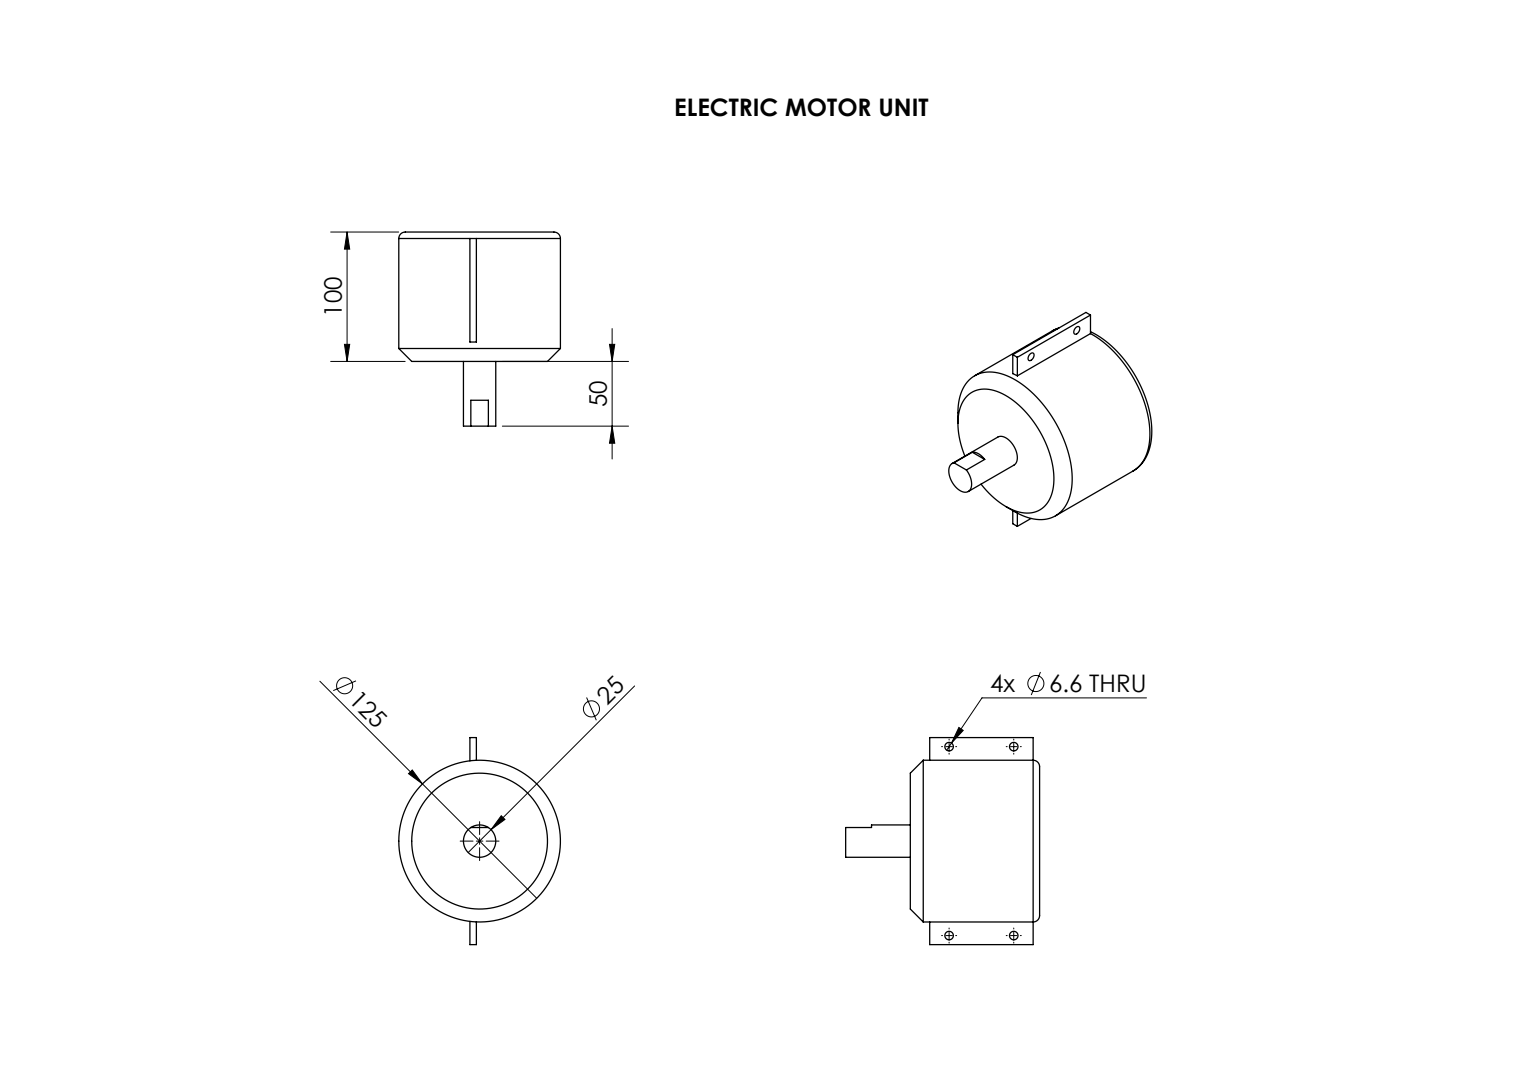
ISO-10303-21;
HEADER;
FILE_DESCRIPTION (('STEP AP214'),
    '1' );
FILE_NAME ('electric motor unit.step',
    '2026-10-08T09:53:37',
    ( '' ),
    ( '' ),
    'SwSTEP 2.0',
    'SolidWorks 2026',
    '' );
FILE_SCHEMA (( 'AUTOMOTIVE_DESIGN' ));
ENDSEC;

DATA;
#74=ORIENTED_EDGE ( 'NONE', *, *, #31039, .F. ) ;
#103=DIRECTION ( 'NONE',  ( 1.000000000000000000, 0.000000000000000000, 0.000000000000000000 ) ) ;
#302=ADVANCED_FACE ( 'NONE', ( #26021 ), #48946, .F. ) ;
#312=DIRECTION ( 'NONE',  ( 1.000000000000000000, 0.000000000000000000, -0.000000000000000000 ) ) ;
#361=ORIENTED_EDGE ( 'NONE', *, *, #62756, .T. ) ;
#411=EDGE_LOOP ( 'NONE', ( #54319, #60311, #25964, #66217 ) ) ;
#435=ORIENTED_EDGE ( 'NONE', *, *, #50527, .T. ) ;
#592=ORIENTED_EDGE ( 'NONE', *, *, #52648, .T. ) ;
#701=DIRECTION ( 'NONE',  ( -0.000000000000000000, -1.000000000000000000, -0.000000000000000000 ) ) ;
#748=DIRECTION ( 'NONE',  ( -2.628368902995175337E-16, -1.000000000000000000, 0.000000000000000000 ) ) ;
#850=LINE ( 'NONE', #68873, #20942 ) ;
#851=DIRECTION ( 'NONE',  ( 0.000000000000000000, 0.000000000000000000, -1.000000000000000000 ) ) ;
#862=ORIENTED_EDGE ( 'NONE', *, *, #52454, .F. ) ;
#988=ORIENTED_EDGE ( 'NONE', *, *, #17612, .T. ) ;
#1081=EDGE_CURVE ( 'NONE', #58897, #8861, #49235, .T. ) ;
#1100=DIRECTION ( 'NONE',  ( -1.000000000000000000, 0.000000000000000000, 0.000000000000000000 ) ) ;
#1101=ORIENTED_EDGE ( 'NONE', *, *, #21972, .F. ) ;
#1138=ORIENTED_EDGE ( 'NONE', *, *, #48438, .T. ) ;
#1246=VERTEX_POINT ( 'NONE', #31110 ) ;
#1350=CIRCLE ( 'NONE', #16923, 3.299999999999997158 ) ;
#1373=AXIS2_PLACEMENT_3D ( 'NONE', #24818, #13162, #19174 ) ;
#1428=EDGE_CURVE ( 'NONE', #19508, #17352, #18011, .T. ) ;
#1449=CARTESIAN_POINT ( 'NONE',  ( -57.50000000000000000, 0.000000000000000000, -270.0000000000000000 ) ) ;
#1479=FACE_OUTER_BOUND ( 'NONE', #30990, .T. ) ;
#1540=ORIENTED_EDGE ( 'NONE', *, *, #59533, .T. ) ;
#1570=CIRCLE ( 'NONE', #60360, 3.299999999999997158 ) ;
#1692=SURFACE_STYLE_FILL_AREA ( #25327 ) ;
#1812=DIRECTION ( 'NONE',  ( -1.000000000000000000, 0.000000000000000000, 0.000000000000000000 ) ) ;
#1846=CARTESIAN_POINT ( 'NONE',  ( -7.500000000000015099, -73.00000000000001421, -204.9999999999999716 ) ) ;
#1897=APPLICATION_CONTEXT ( 'automotive_design' ) ;
#1914=DIRECTION ( 'NONE',  ( 0.000000000000000000, -1.000000000000000000, 0.000000000000000000 ) ) ;
#1941=TOROIDAL_SURFACE ( 'NONE', #16270, 57.50000000000000000, 5.000000000000000000 ) ;
#2035=CLOSED_SHELL ( 'NONE', ( #30843, #53299, #302, #25026, #60112, #57640, #40573, #22486, #44929, #51198, #42095, #58290, #61829, #7482, #45373, #47263, #49888, #8489, #25397, #17549, #53469, #11560, #6297, #37604, #32650, #6641, #53402, #33495, #63872, #73659, #3012 ) ) ;
#2196=ORIENTED_EDGE ( 'NONE', *, *, #1428, .T. ) ;
#2277=ORIENTED_EDGE ( 'NONE', *, *, #3250, .T. ) ;
#2728=COLOUR_RGB ( '', 0.72549020, 0.75294118, 0.79215686) ;
#2822=DIRECTION ( 'NONE',  ( 1.000000000000000000, 0.000000000000000000, -0.000000000000000000 ) ) ;
#2995=ORIENTED_EDGE ( 'NONE', *, *, #17255, .F. ) ;
#3012=ADVANCED_FACE ( 'NONE', ( #22118 ), #14704, .F. ) ;
#3047=CARTESIAN_POINT ( 'NONE',  ( -2.500000000000015543, -73.00000000000001421, -255.0000000000000000 ) ) ;
#3250=EDGE_CURVE ( 'NONE', #46252, #45911, #14903, .T. ) ;
#3266=LINE ( 'NONE', #71272, #46651 ) ;
#3360=EDGE_CURVE ( 'NONE', #56357, #68556, #30997, .T. ) ;
#3614=ORIENTED_EDGE ( 'NONE', *, *, #35996, .T. ) ;
#3644=DIRECTION ( 'NONE',  ( 3.035766082959412415E-16, 1.000000000000000000, 0.000000000000000000 ) ) ;
#3658=AXIS2_PLACEMENT_3D ( 'NONE', #24375, #64239, #748 ) ;
#3682=CARTESIAN_POINT ( 'NONE',  ( -2.499999999999970690, 73.00000000000001421, -204.9999999999999716 ) ) ;
#3953=LINE ( 'NONE', #26854, #13909 ) ;
#3990=EDGE_CURVE ( 'NONE', #70803, #36870, #41096, .T. ) ;
#4050=DIRECTION ( 'NONE',  ( 1.000000000000000000, -3.035766082959412415E-16, 0.000000000000000000 ) ) ;
#4113=ORIENTED_EDGE ( 'NONE', *, *, #71182, .F. ) ;
#4170=EDGE_LOOP ( 'NONE', ( #2196, #10893 ) ) ;
#4251=ORIENTED_EDGE ( 'NONE', *, *, #46885, .T. ) ;
#4271=AXIS2_PLACEMENT_3D ( 'NONE', #41588, #29553, #64905 ) ;
#4350=ORIENTED_EDGE ( 'NONE', *, *, #62756, .F. ) ;
#4452=DIRECTION ( 'NONE',  ( -1.000000000000000000, 0.000000000000000000, -0.000000000000000000 ) ) ;
#4760=ORIENTED_EDGE ( 'NONE', *, *, #67736, .T. ) ;
#4846=ORIENTED_EDGE ( 'NONE', *, *, #59697, .F. ) ;
#4933=CIRCLE ( 'NONE', #1373, 62.50000000000000000 ) ;
#5052=AXIS2_PLACEMENT_3D ( 'NONE', #1449, #701, #36713 ) ;
#5114=DIRECTION ( 'NONE',  ( -3.035766082959412415E-16, -1.000000000000000000, -0.000000000000000000 ) ) ;
#5250=DIRECTION ( 'NONE',  ( -2.628368902995175337E-16, -1.000000000000000000, 0.000000000000000000 ) ) ;
#5361=AXIS2_PLACEMENT_3D ( 'NONE', #22738, #45676, #15965 ) ;
#5589=ORIENTED_EDGE ( 'NONE', *, *, #60526, .F. ) ;
#5681=DIRECTION ( 'NONE',  ( -2.628368902995175337E-16, -1.000000000000000000, 0.000000000000000000 ) ) ;
#5695=CARTESIAN_POINT ( 'NONE',  ( 62.50000000000000000, 0.000000000000000000, -184.9999999999999432 ) ) ;
#5706=FACE_OUTER_BOUND ( 'NONE', #38771, .T. ) ;
#5826=ORIENTED_EDGE ( 'NONE', *, *, #18491, .F. ) ;
#5919=FACE_OUTER_BOUND ( 'NONE', #16578, .T. ) ;
#5929=CARTESIAN_POINT ( 'NONE',  ( -62.50000000000000000, 7.654042494670957804E-15, -270.0000000000000000 ) ) ;
#6030=CARTESIAN_POINT ( 'NONE',  ( -7.500000000000015987, -76.30000000000001137, -204.9999999999999716 ) ) ;
#6194=LINE ( 'NONE', #16347, #44271 ) ;
#6210=VECTOR ( 'NONE', #10753, 1000.000000000000000 ) ;
#6241=DIRECTION ( 'NONE',  ( -1.000000000000000000, 0.000000000000000000, 0.000000000000000000 ) ) ;
#6297=ADVANCED_FACE ( 'NONE', ( #11593, #45473, #34534 ), #69492, .F. ) ;
#6395=CARTESIAN_POINT ( 'NONE',  ( -7.499999999999969802, 73.00000000000001421, -255.0000000000000000 ) ) ;
#6475=AXIS2_PLACEMENT_3D ( 'NONE', #28429, #40094, #32948 ) ;
#6550=CARTESIAN_POINT ( 'NONE',  ( 0.000000000000000000, 0.000000000000000000, -175.0000000000000000 ) ) ;
#6641=ADVANCED_FACE ( 'NONE', ( #72072, #33318, #39359 ), #21297, .T. ) ;
#6670=ORIENTED_EDGE ( 'NONE', *, *, #21705, .F. ) ;
#6743=EDGE_LOOP ( 'NONE', ( #46150, #36857 ) ) ;
#6818=DIRECTION ( 'NONE',  ( -1.000000000000000000, 0.000000000000000000, 0.000000000000000000 ) ) ;
#6845=EDGE_LOOP ( 'NONE', ( #46434, #7193 ) ) ;
#6891=CARTESIAN_POINT ( 'NONE',  ( -2.499999999999971578, 69.70000000000003126, -255.0000000000000000 ) ) ;
#7095=CIRCLE ( 'NONE', #23904, 3.299999999999983391 ) ;
#7161=AXIS2_PLACEMENT_3D ( 'NONE', #73193, #26956, #72082 ) ;
#7193=ORIENTED_EDGE ( 'NONE', *, *, #65149, .F. ) ;
#7283=AXIS2_PLACEMENT_3D ( 'NONE', #60970, #33494, #43696 ) ;
#7344=ORIENTED_EDGE ( 'NONE', *, *, #3250, .F. ) ;
#7449=DIRECTION ( 'NONE',  ( 1.000000000000000000, -3.061616997868382648E-16, -0.000000000000000000 ) ) ;
#7454=EDGE_CURVE ( 'NONE', #45911, #54824, #40915, .T. ) ;
#7482=ADVANCED_FACE ( 'NONE', ( #29600 ), #35312, .T. ) ;
#7679=LINE ( 'NONE', #53542, #74290 ) ;
#7748=VECTOR ( 'NONE', #42150, 1000.000000000000000 ) ;
#7797=CARTESIAN_POINT ( 'NONE',  ( -7.500000000000016875, -80.00000000000001421, -189.9999999999999147 ) ) ;
#7814=CARTESIAN_POINT ( 'NONE',  ( 6.782329983125270800, 10.49999999999999467, -145.0000000000000000 ) ) ;
#8026=SURFACE_SIDE_STYLE ('',( #1692 ) ) ;
#8037=AXIS2_PLACEMENT_3D ( 'NONE', #58333, #54183, #31232 ) ;
#8162=DIRECTION ( 'NONE',  ( -0.000000000000000000, -0.000000000000000000, -1.000000000000000000 ) ) ;
#8300=DIRECTION ( 'NONE',  ( 0.000000000000000000, 0.000000000000000000, -1.000000000000000000 ) ) ;
#8418=ORIENTED_EDGE ( 'NONE', *, *, #21972, .T. ) ;
#8489=ADVANCED_FACE ( 'NONE', ( #31932 ), #60891, .F. ) ;
#8518=CIRCLE ( 'NONE', #44539, 3.299999999999983391 ) ;
#8603=( NAMED_UNIT ( * ) SI_UNIT ( $, .STERADIAN. ) SOLID_ANGLE_UNIT ( ) );
#8735=EDGE_CURVE ( 'NONE', #28195, #41791, #63793, .T. ) ;
#8755=EDGE_CURVE ( 'NONE', #43515, #60602, #68396, .T. ) ;
#8796=LINE ( 'NONE', #31713, #23348 ) ;
#8861=VERTEX_POINT ( 'NONE', #69850 ) ;
#8895=CARTESIAN_POINT ( 'NONE',  ( -7.499999999999969802, 76.30000000000001137, -204.9999999999999716 ) ) ;
#8926=CARTESIAN_POINT ( 'NONE',  ( -7.500000000000011546, -62.04836822995428491, -270.0000000000000000 ) ) ;
#8965=( NAMED_UNIT ( * ) SI_UNIT ( $, .STERADIAN. ) SOLID_ANGLE_UNIT ( ) );
#9003=VECTOR ( 'NONE', #20553, 1000.000000000000000 ) ;
#9296=ORIENTED_EDGE ( 'NONE', *, *, #25138, .F. ) ;
#9298=CYLINDRICAL_SURFACE ( 'NONE', #7161, 3.299999999999983391 ) ;
#9305=CARTESIAN_POINT ( 'NONE',  ( -7.500000000000015987, -76.29999999999999716, -255.0000000000000000 ) ) ;
#9325=SHAPE_REPRESENTATION_RELATIONSHIP ( 'NONE' , 'NONE' ,  #72820, #21132 ) ;
#9442=LINE ( 'NONE', #19610, #22727 ) ;
#9750=DIRECTION ( 'NONE',  ( -0.7071067811865485719, 0.000000000000000000, -0.7071067811865465735 ) ) ;
#9822=ORIENTED_EDGE ( 'NONE', *, *, #23184, .T. ) ;
#9848=AXIS2_PLACEMENT_3D ( 'NONE', #39904, #17697, #63579 ) ;
#10049=CARTESIAN_POINT ( 'NONE',  ( 0.000000000000000000, 0.000000000000000000, -275.0000000000000000 ) ) ;
#10147=ORIENTED_EDGE ( 'NONE', *, *, #43144, .F. ) ;
#10415=ORIENTED_EDGE ( 'NONE', *, *, #54147, .T. ) ;
#10450=CIRCLE ( 'NONE', #8037, 52.50000000000002132 ) ;
#10569=FACE_OUTER_BOUND ( 'NONE', #62660, .T. ) ;
#10575=VECTOR ( 'NONE', #5114, 1000.000000000000000 ) ;
#10601=AXIS2_PLACEMENT_3D ( 'NONE', #13781, #59665, #20550 ) ;
#10656=CARTESIAN_POINT ( 'NONE',  ( 12.49999999999999645, 0.000000000000000000, -175.0000000000000000 ) ) ;
#10753=DIRECTION ( 'NONE',  ( -0.000000000000000000, -0.000000000000000000, 1.000000000000000000 ) ) ;
#10867=UNCERTAINTY_MEASURE_WITH_UNIT (LENGTH_MEASURE( 1.000000000000000082E-05 ), #72476, 'distance_accuracy_value', 'NONE');
#10893=ORIENTED_EDGE ( 'NONE', *, *, #27823, .T. ) ;
#10996=PLANE ( 'NONE',  #14198 ) ;
#11029=CIRCLE ( 'NONE', #18269, 3.299999999999997158 ) ;
#11050=ORIENTED_EDGE ( 'NONE', *, *, #64960, .F. ) ;
#11195=DIRECTION ( 'NONE',  ( 2.628368902995164490E-16, 1.000000000000000000, 0.000000000000000000 ) ) ;
#11360=EDGE_CURVE ( 'NONE', #60498, #28566, #43303, .T. ) ;
#11393=ORIENTED_EDGE ( 'NONE', *, *, #11360, .F. ) ;
#11528=CARTESIAN_POINT ( 'NONE',  ( 0.000000000000000000, 0.000000000000000000, -275.0000000000000000 ) ) ;
#11552=DIRECTION ( 'NONE',  ( 1.000000000000000000, -3.061616997868382648E-16, -0.000000000000000000 ) ) ;
#11560=ADVANCED_FACE ( 'NONE', ( #26385, #43337, #10569 ), #49312, .T. ) ;
#11575=CARTESIAN_POINT ( 'NONE',  ( -62.50000000000000000, 7.654042494670957804E-15, -184.9999999999999432 ) ) ;
#11593=FACE_BOUND ( 'NONE', #62231, .T. ) ;
#11635=ORIENTED_EDGE ( 'NONE', *, *, #12276, .T. ) ;
#11806=EDGE_CURVE ( 'NONE', #65637, #48516, #4933, .T. ) ;
#11844=FACE_OUTER_BOUND ( 'NONE', #29116, .T. ) ;
#11924=VECTOR ( 'NONE', #71334, 1000.000000000000000 ) ;
#12094=ORIENTED_EDGE ( 'NONE', *, *, #7454, .T. ) ;
#12148=CARTESIAN_POINT ( 'NONE',  ( -7.500000000000015099, -73.00000000000001421, -204.9999999999999716 ) ) ;
#12276=EDGE_CURVE ( 'NONE', #59175, #17352, #47770, .T. ) ;
#12340=DIRECTION ( 'NONE',  ( 2.628368902995164490E-16, 1.000000000000000000, 0.000000000000000000 ) ) ;
#12550=( NAMED_UNIT ( * ) PLANE_ANGLE_UNIT ( ) SI_UNIT ( $, .RADIAN. ) );
#12573=ORIENTED_EDGE ( 'NONE', *, *, #1081, .F. ) ;
#12621=AXIS2_PLACEMENT_3D ( 'NONE', #51765, #58509, #312 ) ;
#12671=ORIENTED_EDGE ( 'NONE', *, *, #16152, .T. ) ;
#12691=CARTESIAN_POINT ( 'NONE',  ( 0.000000000000000000, 0.000000000000000000, -184.9999999999999432 ) ) ;
#13153=AXIS2_PLACEMENT_3D ( 'NONE', #24806, #70649, #37211 ) ;
#13162=DIRECTION ( 'NONE',  ( -0.000000000000000000, -0.000000000000000000, -1.000000000000000000 ) ) ;
#13218=EDGE_CURVE ( 'NONE', #20502, #14677, #59869, .T. ) ;
#13293=( LENGTH_UNIT ( ) NAMED_UNIT ( * ) SI_UNIT ( .MILLI., .METRE. ) );
#13320=CARTESIAN_POINT ( 'NONE',  ( -2.500000000000014655, -69.70000000000003126, -255.0000000000000000 ) ) ;
#13374=AXIS2_PLACEMENT_3D ( 'NONE', #55982, #49591, #26291 ) ;
#13556=LINE ( 'NONE', #36861, #7748 ) ;
#13587=AXIS2_PLACEMENT_3D ( 'NONE', #45939, #69592, #33899 ) ;
#13620=ORIENTED_EDGE ( 'NONE', *, *, #17255, .T. ) ;
#13781=CARTESIAN_POINT ( 'NONE',  ( 0.000000000000000000, 0.000000000000000000, -270.0000000000000000 ) ) ;
#13845=AXIS2_PLACEMENT_3D ( 'NONE', #10049, #14577, #38252 ) ;
#13848=SURFACE_STYLE_FILL_AREA ( #72108 ) ;
#13872=ORIENTED_EDGE ( 'NONE', *, *, #25138, .T. ) ;
#13909=VECTOR ( 'NONE', #27211, 1000.000000000000000 ) ;
#14112=ORIENTED_EDGE ( 'NONE', *, *, #31568, .F. ) ;
#14114=AXIS2_PLACEMENT_3D ( 'NONE', #66883, #60158, #31549 ) ;
#14129=ORIENTED_EDGE ( 'NONE', *, *, #52454, .T. ) ;
#14164=ORIENTED_EDGE ( 'NONE', *, *, #1081, .T. ) ;
#14198=AXIS2_PLACEMENT_3D ( 'NONE', #21899, #33168, #16258 ) ;
#14261=PLANE ( 'NONE',  #13153 ) ;
#14402=PLANE ( 'NONE',  #69131 ) ;
#14414=ORIENTED_EDGE ( 'NONE', *, *, #46092, .T. ) ;
#14577=DIRECTION ( 'NONE',  ( 0.000000000000000000, 0.000000000000000000, -1.000000000000000000 ) ) ;
#14677=VERTEX_POINT ( 'NONE', #49938 ) ;
#14704=CYLINDRICAL_SURFACE ( 'NONE', #27337, 3.299999999999983391 ) ;
#14826=CARTESIAN_POINT ( 'NONE',  ( 0.000000000000000000, 0.000000000000000000, -270.0000000000000000 ) ) ;
#14903=LINE ( 'NONE', #54027, #59829 ) ;
#14969=CARTESIAN_POINT ( 'NONE',  ( -7.500000000000016875, -80.00000000000001421, -189.9999999999999147 ) ) ;
#15362=ORIENTED_EDGE ( 'NONE', *, *, #21277, .F. ) ;
#15420=ORIENTED_EDGE ( 'NONE', *, *, #53796, .F. ) ;
#15467=CYLINDRICAL_SURFACE ( 'NONE', #47896, 12.49999999999999645 ) ;
#15499=VERTEX_POINT ( 'NONE', #5929 ) ;
#15513=ORIENTED_EDGE ( 'NONE', *, *, #64442, .T. ) ;
#15807=CIRCLE ( 'NONE', #9848, 12.49999999999999645 ) ;
#15965=DIRECTION ( 'NONE',  ( -1.000000000000000000, 0.000000000000000000, 0.000000000000000000 ) ) ;
#16108=VERTEX_POINT ( 'NONE', #29746 ) ;
#16152=EDGE_CURVE ( 'NONE', #41791, #67978, #53077, .T. ) ;
#16239=ORIENTED_EDGE ( 'NONE', *, *, #8755, .F. ) ;
#16252=ORIENTED_EDGE ( 'NONE', *, *, #45421, .T. ) ;
#16258=DIRECTION ( 'NONE',  ( 3.035766082959412415E-16, 1.000000000000000000, 0.000000000000000000 ) ) ;
#16270=AXIS2_PLACEMENT_3D ( 'NONE', #58457, #64118, #6241 ) ;
#16310=MECHANICAL_DESIGN_GEOMETRIC_PRESENTATION_REPRESENTATION('',(#28319),#59517);
#16347=CARTESIAN_POINT ( 'NONE',  ( -7.499999999999968914, 79.99999999999998579, -269.9999999999999432 ) ) ;
#16355=EDGE_LOOP ( 'NONE', ( #22088, #592, #74262, #11050 ) ) ;
#16369=CARTESIAN_POINT ( 'NONE',  ( -2.500000000000017319, -80.00000000000001421, -269.9999999999999432 ) ) ;
#16373=DIRECTION ( 'NONE',  ( -2.628368902995175337E-16, -1.000000000000000000, 0.000000000000000000 ) ) ;
#16391=CARTESIAN_POINT ( 'NONE',  ( -62.50000000000000000, 7.654042494670957804E-15, -275.0000000000000000 ) ) ;
#16486=ORIENTED_EDGE ( 'NONE', *, *, #59697, .T. ) ;
#16494=ORIENTED_EDGE ( 'NONE', *, *, #19258, .T. ) ;
#16557=VERTEX_POINT ( 'NONE', #53348 ) ;
#16578=EDGE_LOOP ( 'NONE', ( #54271, #65011, #23966, #27736, #3614, #65107, #26363, #21177 ) ) ;
#16725=ORIENTED_EDGE ( 'NONE', *, *, #57755, .T. ) ;
#16923=AXIS2_PLACEMENT_3D ( 'NONE', #3682, #71692, #26944 ) ;
#17255=EDGE_CURVE ( 'NONE', #67978, #16108, #38669, .T. ) ;
#17304=AXIS2_PLACEMENT_3D ( 'NONE', #37039, #72353, #36289 ) ;
#17339=CYLINDRICAL_SURFACE ( 'NONE', #25457, 62.50000000000000000 ) ;
#17347=DIRECTION ( 'NONE',  ( -1.000000000000000000, -3.907985046680551022E-14, 0.000000000000000000 ) ) ;
#17352=VERTEX_POINT ( 'NONE', #68636 ) ;
#17357=DIRECTION ( 'NONE',  ( -3.035766082959412415E-16, -1.000000000000000000, -0.000000000000000000 ) ) ;
#17395=PRODUCT_CONTEXT ( 'NONE', #29621, 'mechanical' ) ;
#17544=CYLINDRICAL_SURFACE ( 'NONE', #66014, 62.50000000000000000 ) ;
#17549=ADVANCED_FACE ( 'NONE', ( #25353 ), #43406, .F. ) ;
#17612=EDGE_CURVE ( 'NONE', #28566, #28744, #8796, .T. ) ;
#17697=DIRECTION ( 'NONE',  ( 0.000000000000000000, 0.000000000000000000, 1.000000000000000000 ) ) ;
#17702=VECTOR ( 'NONE', #44493, 1000.000000000000000 ) ;
#17760=CARTESIAN_POINT ( 'NONE',  ( 0.000000000000000000, 0.000000000000000000, -189.9999999999999147 ) ) ;
#17773=CARTESIAN_POINT ( 'NONE',  ( -7.499999999999968914, 79.99999999999998579, -189.9999999999999147 ) ) ;
#17824=CARTESIAN_POINT ( 'NONE',  ( -2.499999999999974243, 62.44997998398397954, -275.0000000000000000 ) ) ;
#17827=CIRCLE ( 'NONE', #27423, 62.50000000000000000 ) ;
#17921=FACE_OUTER_BOUND ( 'NONE', #31873, .T. ) ;
#18011=CIRCLE ( 'NONE', #51603, 57.50000000000000000 ) ;
#18018=VECTOR ( 'NONE', #8300, 1000.000000000000000 ) ;
#18112=CARTESIAN_POINT ( 'NONE',  ( -7.500000000000015099, -73.00000000000001421, -255.0000000000000000 ) ) ;
#18269=AXIS2_PLACEMENT_3D ( 'NONE', #54497, #19534, #42486 ) ;
#18314=AXIS2_PLACEMENT_3D ( 'NONE', #14826, #32111, #42668 ) ;
#18316=DIRECTION ( 'NONE',  ( -0.000000000000000000, -0.000000000000000000, 1.000000000000000000 ) ) ;
#18420=ORIENTED_EDGE ( 'NONE', *, *, #67960, .T. ) ;
#18491=EDGE_CURVE ( 'NONE', #1246, #39261, #44228, .T. ) ;
#18590=LINE ( 'NONE', #23500, #22811 ) ;
#18630=AXIS2_PLACEMENT_3D ( 'NONE', #73390, #66658, #73011 ) ;
#18638=VECTOR ( 'NONE', #66465, 1000.000000000000000 ) ;
#18647=CYLINDRICAL_SURFACE ( 'NONE', #4271, 3.299999999999997158 ) ;
#18827=CARTESIAN_POINT ( 'NONE',  ( -2.500000000000017319, -80.00000000000001421, -189.9999999999999147 ) ) ;
#18845=VECTOR ( 'NONE', #9750, 1000.000000000000000 ) ;
#18974=EDGE_LOOP ( 'NONE', ( #57902, #37363, #12573, #43298 ) ) ;
#19154=CARTESIAN_POINT ( 'NONE',  ( -6.782329983125270800, 10.49999999999999467, -145.0000000000000000 ) ) ;
#19174=DIRECTION ( 'NONE',  ( -1.000000000000000000, 0.000000000000000000, 0.000000000000000000 ) ) ;
#19206=LINE ( 'NONE', #59813, #18018 ) ;
#19258=EDGE_CURVE ( 'NONE', #45911, #70771, #63294, .T. ) ;
#19508=VERTEX_POINT ( 'NONE', #42434 ) ;
#19534=DIRECTION ( 'NONE',  ( -1.000000000000000000, 3.061616997868382648E-16, 0.000000000000000000 ) ) ;
#19555=DIRECTION ( 'NONE',  ( -1.000000000000000000, 3.061616997868382648E-16, 0.000000000000000000 ) ) ;
#19573=ORIENTED_EDGE ( 'NONE', *, *, #23372, .F. ) ;
#19610=CARTESIAN_POINT ( 'NONE',  ( -7.499999999999969802, 76.30000000000001137, -204.9999999999999716 ) ) ;
#19636=CARTESIAN_POINT ( 'NONE',  ( -2.499999999999970690, 73.00000000000001421, -255.0000000000000000 ) ) ;
#19735=DIRECTION ( 'NONE',  ( 1.000000000000000000, 0.000000000000000000, 0.000000000000000000 ) ) ;
#19847=ORIENTED_EDGE ( 'NONE', *, *, #63123, .F. ) ;
#20050=VERTEX_POINT ( 'NONE', #52720 ) ;
#20152=CARTESIAN_POINT ( 'NONE',  ( -2.500000000000011990, -62.44997998398397954, -269.9999999999999432 ) ) ;
#20172=ORIENTED_EDGE ( 'NONE', *, *, #54847, .T. ) ;
#20393=DIRECTION ( 'NONE',  ( 1.000000000000000000, -3.061616997868382648E-16, -0.000000000000000000 ) ) ;
#20502=VERTEX_POINT ( 'NONE', #52529 ) ;
#20550=DIRECTION ( 'NONE',  ( -1.000000000000000000, 0.000000000000000000, 0.000000000000000000 ) ) ;
#20553=DIRECTION ( 'NONE',  ( -0.000000000000000000, -0.000000000000000000, 1.000000000000000000 ) ) ;
#20568=ORIENTED_EDGE ( 'NONE', *, *, #3990, .T. ) ;
#20596=LINE ( 'NONE', #43547, #18638 ) ;
#20796=EDGE_CURVE ( 'NONE', #15499, #65637, #67901, .T. ) ;
#20847=CIRCLE ( 'NONE', #6475, 62.50000000000000000 ) ;
#20942=VECTOR ( 'NONE', #17357, 1000.000000000000000 ) ;
#21132=ADVANCED_BREP_SHAPE_REPRESENTATION ( '', ( #37419, #43395 ), #41132 ) ;
#21177=ORIENTED_EDGE ( 'NONE', *, *, #50081, .T. ) ;
#21277=EDGE_CURVE ( 'NONE', #20050, #32222, #11029, .T. ) ;
#21297=PLANE ( 'NONE',  #56843 ) ;
#21436=ORIENTED_EDGE ( 'NONE', *, *, #54640, .F. ) ;
#21442=LINE ( 'NONE', #73322, #49807 ) ;
#21668=EDGE_CURVE ( 'NONE', #15499, #56357, #68728, .T. ) ;
#21673=FACE_BOUND ( 'NONE', #25864, .T. ) ;
#21702=AXIS2_PLACEMENT_3D ( 'NONE', #19154, #1914, #58641 ) ;
#21705=EDGE_CURVE ( 'NONE', #59850, #48671, #1570, .T. ) ;
#21786=PRODUCT_DEFINITION_SHAPE ( 'NONE', 'NONE',  #33419 ) ;
#21797=CIRCLE ( 'NONE', #48215, 3.299999999999997158 ) ;
#21899=CARTESIAN_POINT ( 'NONE',  ( -7.499999999999992895, 2.289750019674042456E-15, 0.000000000000000000 ) ) ;
#21972=EDGE_CURVE ( 'NONE', #41089, #33185, #21797, .T. ) ;
#21988=LINE ( 'NONE', #17824, #44781 ) ;
#21996=EDGE_CURVE ( 'NONE', #16108, #67978, #43405, .T. ) ;
#22060=CARTESIAN_POINT ( 'NONE',  ( -2.499999999999992895, 7.589415207398510330E-16, 0.000000000000000000 ) ) ;
#22088=ORIENTED_EDGE ( 'NONE', *, *, #21705, .T. ) ;
#22118=FACE_OUTER_BOUND ( 'NONE', #46049, .T. ) ;
#22371=ORIENTED_EDGE ( 'NONE', *, *, #42422, .F. ) ;
#22486=ADVANCED_FACE ( 'NONE', ( #5706 ), #17339, .T. ) ;
#22649=FACE_OUTER_BOUND ( 'NONE', #60918, .T. ) ;
#22705=ORIENTED_EDGE ( 'NONE', *, *, #37349, .F. ) ;
#22727=VECTOR ( 'NONE', #31998, 1000.000000000000000 ) ;
#22738=CARTESIAN_POINT ( 'NONE',  ( 0.000000000000000000, 0.000000000000000000, -184.9999999999999432 ) ) ;
#22799=CARTESIAN_POINT ( 'NONE',  ( -7.500000000000014211, -69.70000000000001705, -204.9999999999999716 ) ) ;
#22811=VECTOR ( 'NONE', #46813, 1000.000000000000000 ) ;
#22862=CYLINDRICAL_SURFACE ( 'NONE', #37805, 3.299999999999997158 ) ;
#22866=EDGE_CURVE ( 'NONE', #60498, #65293, #35637, .T. ) ;
#23017=VECTOR ( 'NONE', #3644, 1000.000000000000000 ) ;
#23019=CARTESIAN_POINT ( 'NONE',  ( 0.000000000000000000, 0.000000000000000000, -125.0000000000000000 ) ) ;
#23184=EDGE_CURVE ( 'NONE', #71821, #24035, #55552, .T. ) ;
#23348=VECTOR ( 'NONE', #54658, 1000.000000000000000 ) ;
#23372=EDGE_CURVE ( 'NONE', #40539, #62152, #21988, .T. ) ;
#23380=CIRCLE ( 'NONE', #59436, 12.49999999999999645 ) ;
#23489=VERTEX_POINT ( 'NONE', #28735 ) ;
#23500=CARTESIAN_POINT ( 'NONE',  ( 62.50000000000000000, 7.654042494670957804E-15, -184.9999999999999432 ) ) ;
#23523=DIRECTION ( 'NONE',  ( 0.000000000000000000, 0.000000000000000000, -1.000000000000000000 ) ) ;
#23728=ORIENTED_EDGE ( 'NONE', *, *, #73905, .T. ) ;
#23904=AXIS2_PLACEMENT_3D ( 'NONE', #3047, #19555, #65072 ) ;
#23939=PLANE ( 'NONE',  #12621 ) ;
#23966=ORIENTED_EDGE ( 'NONE', *, *, #45421, .F. ) ;
#24035=VERTEX_POINT ( 'NONE', #43189 ) ;
#24075=DIRECTION ( 'NONE',  ( -1.000000000000000000, 0.000000000000000000, 0.000000000000000000 ) ) ;
#24215=DIRECTION ( 'NONE',  ( 0.000000000000000000, 0.000000000000000000, -1.000000000000000000 ) ) ;
#24375=CARTESIAN_POINT ( 'NONE',  ( -2.500000000000015543, -73.00000000000001421, -255.0000000000000000 ) ) ;
#24537=CARTESIAN_POINT ( 'NONE',  ( -7.499999999999970690, 69.70000000000003126, -255.0000000000000000 ) ) ;
#24770=LINE ( 'NONE', #53711, #26325 ) ;
#24806=CARTESIAN_POINT ( 'NONE',  ( -7.500000000000016875, -80.00000000000001421, -269.9999999999999432 ) ) ;
#24818=CARTESIAN_POINT ( 'NONE',  ( 0.000000000000000000, 0.000000000000000000, -184.9999999999999432 ) ) ;
#24821=LINE ( 'NONE', #64679, #73542 ) ;
#24907=DIRECTION ( 'NONE',  ( -1.000000000000000000, 0.000000000000000000, 0.000000000000000000 ) ) ;
#24967=ORIENTED_EDGE ( 'NONE', *, *, #46092, .F. ) ;
#25026=ADVANCED_FACE ( 'NONE', ( #30405 ), #41335, .F. ) ;
#25138=EDGE_CURVE ( 'NONE', #59175, #40539, #65382, .T. ) ;
#25158=CARTESIAN_POINT ( 'NONE',  ( 0.000000000000000000, 0.000000000000000000, -270.0000000000000000 ) ) ;
#25327=FILL_AREA_STYLE ('',( #59915 ) ) ;
#25353=FACE_OUTER_BOUND ( 'NONE', #32700, .T. ) ;
#25397=ADVANCED_FACE ( 'NONE', ( #40140 ), #22862, .F. ) ;
#25457=AXIS2_PLACEMENT_3D ( 'NONE', #28604, #63591, #103 ) ;
#25565=UNCERTAINTY_MEASURE_WITH_UNIT (LENGTH_MEASURE( 1.000000000000000082E-05 ), #13293, 'distance_accuracy_value', 'NONE');
#25708=DIRECTION ( 'NONE',  ( 0.000000000000000000, 0.000000000000000000, 1.000000000000000000 ) ) ;
#25752=DIRECTION ( 'NONE',  ( 3.035766082959412415E-16, 1.000000000000000000, 0.000000000000000000 ) ) ;
#25800=CARTESIAN_POINT ( 'NONE',  ( -7.500000000000016875, -80.00000000000001421, -189.9999999999999147 ) ) ;
#25845=PRODUCT_DEFINITION_CONTEXT ( 'detailed design', #1897, 'design' ) ;
#25864=EDGE_LOOP ( 'NONE', ( #26166, #16725 ) ) ;
#25880=SURFACE_STYLE_USAGE ( .BOTH. , #37913 ) ;
#25964=ORIENTED_EDGE ( 'NONE', *, *, #42422, .T. ) ;
#26021=FACE_OUTER_BOUND ( 'NONE', #16355, .T. ) ;
#26089=AXIS2_PLACEMENT_3D ( 'NONE', #37500, #32939, #49863 ) ;
#26166=ORIENTED_EDGE ( 'NONE', *, *, #11360, .T. ) ;
#26254=ORIENTED_EDGE ( 'NONE', *, *, #72617, .F. ) ;
#26291=DIRECTION ( 'NONE',  ( 2.628368902995175337E-16, 1.000000000000000000, 0.000000000000000000 ) ) ;
#26325=VECTOR ( 'NONE', #30763, 1000.000000000000000 ) ;
#26363=ORIENTED_EDGE ( 'NONE', *, *, #58415, .T. ) ;
#26385=FACE_BOUND ( 'NONE', #29466, .T. ) ;
#26431=CIRCLE ( 'NONE', #63646, 3.299999999999983391 ) ;
#26613=PLANE ( 'NONE',  #41903 ) ;
#26652=EDGE_LOOP ( 'NONE', ( #37636, #43197, #7344, #55793 ) ) ;
#26697=ORIENTED_EDGE ( 'NONE', *, *, #46618, .T. ) ;
#26854=CARTESIAN_POINT ( 'NONE',  ( -7.500000000000014211, -69.70000000000003126, -255.0000000000000000 ) ) ;
#26921=DIRECTION ( 'NONE',  ( -1.000000000000000000, 0.000000000000000000, 0.000000000000000000 ) ) ;
#26944=DIRECTION ( 'NONE',  ( -2.628368902995164490E-16, -1.000000000000000000, 0.000000000000000000 ) ) ;
#26956=DIRECTION ( 'NONE',  ( 1.000000000000000000, -3.061616997868382648E-16, -0.000000000000000000 ) ) ;
#27053=EDGE_LOOP ( 'NONE', ( #4251, #32061 ) ) ;
#27108=AXIS2_PLACEMENT_3D ( 'NONE', #23019, #851, #45948 ) ;
#27148=PLANE ( 'NONE',  #18630 ) ;
#27211=DIRECTION ( 'NONE',  ( 1.000000000000000000, -3.061616997868382648E-16, -0.000000000000000000 ) ) ;
#27329=FACE_OUTER_BOUND ( 'NONE', #4170, .T. ) ;
#27337=AXIS2_PLACEMENT_3D ( 'NONE', #54930, #27756, #50303 ) ;
#27374=ORIENTED_EDGE ( 'NONE', *, *, #11806, .F. ) ;
#27423=AXIS2_PLACEMENT_3D ( 'NONE', #45937, #68861, #17347 ) ;
#27549=LINE ( 'NONE', #38471, #17702 ) ;
#27736=ORIENTED_EDGE ( 'NONE', *, *, #59261, .F. ) ;
#27756=DIRECTION ( 'NONE',  ( 1.000000000000000000, -3.061616997868382648E-16, -0.000000000000000000 ) ) ;
#27787=CARTESIAN_POINT ( 'NONE',  ( -7.499999999999969802, 73.00000000000001421, -255.0000000000000000 ) ) ;
#27802=CARTESIAN_POINT ( 'NONE',  ( -7.499999999999968914, 79.99999999999998579, -189.9999999999999147 ) ) ;
#27823=EDGE_CURVE ( 'NONE', #17352, #19508, #34525, .T. ) ;
#27977=CARTESIAN_POINT ( 'NONE',  ( -2.500000000000011990, -62.44997998398397954, -275.0000000000000000 ) ) ;
#28016=DIRECTION ( 'NONE',  ( -1.000000000000000000, 1.776356839400250465E-15, 0.000000000000000000 ) ) ;
#28195=VERTEX_POINT ( 'NONE', #33974 ) ;
#28319=STYLED_ITEM ( 'NONE', ( #53891 ), #37419 ) ;
#28346=LINE ( 'NONE', #27977, #43472 ) ;
#28429=CARTESIAN_POINT ( 'NONE',  ( 0.000000000000000000, 0.000000000000000000, -184.9999999999999432 ) ) ;
#28516=DIRECTION ( 'NONE',  ( 1.000000000000000000, -3.061616997868382648E-16, -0.000000000000000000 ) ) ;
#28566=VERTEX_POINT ( 'NONE', #61723 ) ;
#28604=CARTESIAN_POINT ( 'NONE',  ( 0.000000000000000000, 0.000000000000000000, -275.0000000000000000 ) ) ;
#28635=DIRECTION ( 'NONE',  ( -1.000000000000000000, 0.000000000000000000, -0.000000000000000000 ) ) ;
#28735=CARTESIAN_POINT ( 'NONE',  ( -52.50000000000002132, 0.000000000000000000, -175.0000000000000000 ) ) ;
#28744=VERTEX_POINT ( 'NONE', #52286 ) ;
#28774=EDGE_CURVE ( 'NONE', #36870, #60602, #46649, .T. ) ;
#28783=CIRCLE ( 'NONE', #34745, 52.50000000000002132 ) ;
#28903=CARTESIAN_POINT ( 'NONE',  ( 12.49999999999999645, 0.000000000000000000, -175.0000000000000000 ) ) ;
#28955=DIRECTION ( 'NONE',  ( 0.000000000000000000, 0.000000000000000000, -1.000000000000000000 ) ) ;
#29116=EDGE_LOOP ( 'NONE', ( #9296, #11635, #56965, #21436, #24967, #74072 ) ) ;
#29327=ORIENTED_EDGE ( 'NONE', *, *, #35996, .F. ) ;
#29466=EDGE_LOOP ( 'NONE', ( #60592, #13620 ) ) ;
#29553=DIRECTION ( 'NONE',  ( 1.000000000000000000, -3.061616997868382648E-16, -0.000000000000000000 ) ) ;
#29600=FACE_OUTER_BOUND ( 'NONE', #53704, .T. ) ;
#29618=DIRECTION ( 'NONE',  ( 3.035766082959412415E-16, 1.000000000000000000, 0.000000000000000000 ) ) ;
#29621=APPLICATION_CONTEXT ( 'automotive_design' ) ;
#29683=CARTESIAN_POINT ( 'NONE',  ( 12.49999999999999645, 0.000000000000000000, -125.0000000000000000 ) ) ;
#29746=CARTESIAN_POINT ( 'NONE',  ( -2.499999999999969802, 76.29999999999999716, -255.0000000000000000 ) ) ;
#29765=SHAPE_DEFINITION_REPRESENTATION ( #21786, #72820 ) ;
#30194=EDGE_CURVE ( 'NONE', #40539, #40791, #17827, .T. ) ;
#30255=CARTESIAN_POINT ( 'NONE',  ( -7.500000000000016875, -80.00000000000001421, -269.9999999999999432 ) ) ;
#30270=EDGE_CURVE ( 'NONE', #8861, #58897, #7095, .T. ) ;
#30329=AXIS2_PLACEMENT_3D ( 'NONE', #19636, #59507, #47843 ) ;
#30405=FACE_OUTER_BOUND ( 'NONE', #63386, .T. ) ;
#30478=LINE ( 'NONE', #18827, #39541 ) ;
#30502=EDGE_LOOP ( 'NONE', ( #45891, #26697, #62164, #2995 ) ) ;
#30520=VECTOR ( 'NONE', #59680, 1000.000000000000000 ) ;
#30763=DIRECTION ( 'NONE',  ( -0.000000000000000000, -0.000000000000000000, 1.000000000000000000 ) ) ;
#30843=ADVANCED_FACE ( 'NONE', ( #67192 ), #9298, .F. ) ;
#30931=ORIENTED_EDGE ( 'NONE', *, *, #43144, .T. ) ;
#30990=EDGE_LOOP ( 'NONE', ( #1138, #10415 ) ) ;
#30997=CIRCLE ( 'NONE', #10601, 62.50000000000000000 ) ;
#31028=VECTOR ( 'NONE', #52655, 1000.000000000000000 ) ;
#31039=EDGE_CURVE ( 'NONE', #46252, #16557, #48294, .T. ) ;
#31110=CARTESIAN_POINT ( 'NONE',  ( -6.782329983125270800, 10.49999999999999467, -145.0000000000000000 ) ) ;
#31232=DIRECTION ( 'NONE',  ( -1.000000000000000000, 0.000000000000000000, 0.000000000000000000 ) ) ;
#31233=AXIS2_PLACEMENT_3D ( 'NONE', #1846, #7449, #12340 ) ;
#31549=DIRECTION ( 'NONE',  ( -1.000000000000000000, 0.000000000000000000, 0.000000000000000000 ) ) ;
#31568=EDGE_CURVE ( 'NONE', #45157, #65293, #66739, .T. ) ;
#31582=CARTESIAN_POINT ( 'NONE',  ( -2.500000000000017319, -80.00000000000001421, -189.9999999999999147 ) ) ;
#31618=ORIENTED_EDGE ( 'NONE', *, *, #50081, .F. ) ;
#31713=CARTESIAN_POINT ( 'NONE',  ( -12.49999999999999645, 1.530808498934191127E-15, -175.0000000000000000 ) ) ;
#31832=CIRCLE ( 'NONE', #34256, 12.49999999999999645 ) ;
#31833=EDGE_LOOP ( 'NONE', ( #29327, #49092, #19847, #862 ) ) ;
#31836=EDGE_CURVE ( 'NONE', #48671, #59850, #52574, .T. ) ;
#31873=EDGE_LOOP ( 'NONE', ( #74281, #14129, #74, #4350 ) ) ;
#31932=FACE_OUTER_BOUND ( 'NONE', #30502, .T. ) ;
#31984=ORIENTED_EDGE ( 'NONE', *, *, #8735, .T. ) ;
#31998=DIRECTION ( 'NONE',  ( 1.000000000000000000, -3.061616997868382648E-16, -0.000000000000000000 ) ) ;
#32061=ORIENTED_EDGE ( 'NONE', *, *, #21277, .T. ) ;
#32111=DIRECTION ( 'NONE',  ( -0.000000000000000000, -0.000000000000000000, 1.000000000000000000 ) ) ;
#32206=DIRECTION ( 'NONE',  ( 0.000000000000000000, 0.000000000000000000, 1.000000000000000000 ) ) ;
#32222=VERTEX_POINT ( 'NONE', #45312 ) ;
#32365=AXIS2_PLACEMENT_3D ( 'NONE', #35369, #58294, #67821 ) ;
#32582=DIRECTION ( 'NONE',  ( -1.000000000000000000, -1.224646799147354193E-16, 0.000000000000000000 ) ) ;
#32650=ADVANCED_FACE ( 'NONE', ( #61766, #33920, #22649 ), #10996, .F. ) ;
#32700=EDGE_LOOP ( 'NONE', ( #45541, #35509, #70548, #39098 ) ) ;
#32749=DIRECTION ( 'NONE',  ( -0.000000000000000000, -0.000000000000000000, 1.000000000000000000 ) ) ;
#32930=ORIENTED_EDGE ( 'NONE', *, *, #20796, .T. ) ;
#32939=DIRECTION ( 'NONE',  ( 0.000000000000000000, 0.000000000000000000, -1.000000000000000000 ) ) ;
#32948=DIRECTION ( 'NONE',  ( -1.000000000000000000, 0.000000000000000000, 0.000000000000000000 ) ) ;
#33168=DIRECTION ( 'NONE',  ( 1.000000000000000000, -3.035766082959412415E-16, 0.000000000000000000 ) ) ;
#33185=VERTEX_POINT ( 'NONE', #6030 ) ;
#33318=FACE_BOUND ( 'NONE', #27053, .T. ) ;
#33419=PRODUCT_DEFINITION ( 'UNKNOWN', '', #73629, #25845 ) ;
#33439=EDGE_CURVE ( 'NONE', #40791, #53797, #24770, .T. ) ;
#33494=DIRECTION ( 'NONE',  ( 1.000000000000000000, -3.035766082959412415E-16, 0.000000000000000000 ) ) ;
#33495=ADVANCED_FACE ( 'NONE', ( #72104 ), #26613, .F. ) ;
#33630=TOROIDAL_SURFACE ( 'NONE', #37244, 57.50000000000000000, 5.000000000000000000 ) ;
#33684=AXIS2_PLACEMENT_3D ( 'NONE', #49293, #50020, #43315 ) ;
#33863=ORIENTED_EDGE ( 'NONE', *, *, #22866, .T. ) ;
#33899=DIRECTION ( 'NONE',  ( -1.000000000000000000, 0.000000000000000000, -0.000000000000000000 ) ) ;
#33920=FACE_BOUND ( 'NONE', #44055, .T. ) ;
#33974=CARTESIAN_POINT ( 'NONE',  ( -7.499999999999969802, 76.29999999999999716, -255.0000000000000000 ) ) ;
#34034=CARTESIAN_POINT ( 'NONE',  ( 0.000000000000000000, 0.000000000000000000, -270.0000000000000000 ) ) ;
#34110=CARTESIAN_POINT ( 'NONE',  ( -7.499999999999970690, 69.70000000000001705, -204.9999999999999716 ) ) ;
#34256=AXIS2_PLACEMENT_3D ( 'NONE', #51517, #28955, #24075 ) ;
#34317=VECTOR ( 'NONE', #70477, 1000.000000000000000 ) ;
#34525=CIRCLE ( 'NONE', #14114, 57.50000000000000000 ) ;
#34534=FACE_OUTER_BOUND ( 'NONE', #411, .T. ) ;
#34545=VECTOR ( 'NONE', #60629, 1000.000000000000000 ) ;
#34657=DIRECTION ( 'NONE',  ( -2.628368902995175337E-16, -1.000000000000000000, 0.000000000000000000 ) ) ;
#34745=AXIS2_PLACEMENT_3D ( 'NONE', #62270, #56635, #26921 ) ;
#34774=ORIENTED_EDGE ( 'NONE', *, *, #71626, .T. ) ;
#34865=CIRCLE ( 'NONE', #33684, 3.299999999999997158 ) ;
#35094=DIRECTION ( 'NONE',  ( -2.628368902995164490E-16, -1.000000000000000000, 0.000000000000000000 ) ) ;
#35312=CONICAL_SURFACE ( 'NONE', #67735, 62.50000000000000000, 0.7853981633974497223 ) ;
#35322=CARTESIAN_POINT ( 'NONE',  ( -2.499999999999974243, 62.44997998398397954, -189.9999999999999147 ) ) ;
#35369=CARTESIAN_POINT ( 'NONE',  ( 0.000000000000000000, 0.000000000000000000, -189.9999999999999147 ) ) ;
#35382=PLANE ( 'NONE',  #13587 ) ;
#35509=ORIENTED_EDGE ( 'NONE', *, *, #39974, .F. ) ;
#35513=COLOUR_RGB ( '', 0.72549020, 0.75294118, 0.79215686) ;
#35637=LINE ( 'NONE', #28903, #49492 ) ;
#35996=EDGE_CURVE ( 'NONE', #63454, #68556, #28346, .T. ) ;
#36057=DIRECTION ( 'NONE',  ( 1.000000000000000000, -3.061616997868382648E-16, -0.000000000000000000 ) ) ;
#36226=ORIENTED_EDGE ( 'NONE', *, *, #71626, .F. ) ;
#36289=DIRECTION ( 'NONE',  ( -1.000000000000000000, 0.000000000000000000, 0.000000000000000000 ) ) ;
#36489=ORIENTED_EDGE ( 'NONE', *, *, #30270, .T. ) ;
#36522=ORIENTED_EDGE ( 'NONE', *, *, #18491, .T. ) ;
#36656=LINE ( 'NONE', #54694, #34317 ) ;
#36713=DIRECTION ( 'NONE',  ( 0.000000000000000000, 0.000000000000000000, -1.000000000000000000 ) ) ;
#36749=CARTESIAN_POINT ( 'NONE',  ( 0.000000000000000000, 0.000000000000000000, -145.0000000000000000 ) ) ;
#36751=CYLINDRICAL_SURFACE ( 'NONE', #31233, 3.299999999999997158 ) ;
#36857=ORIENTED_EDGE ( 'NONE', *, *, #46618, .F. ) ;
#36861=CARTESIAN_POINT ( 'NONE',  ( -7.499999999999970690, 69.70000000000001705, -204.9999999999999716 ) ) ;
#36870=VERTEX_POINT ( 'NONE', #62032 ) ;
#37039=CARTESIAN_POINT ( 'NONE',  ( 0.000000000000000000, 0.000000000000000000, -125.0000000000000000 ) ) ;
#37095=EDGE_LOOP ( 'NONE', ( #26254, #53334, #27374, #73395 ) ) ;
#37211=DIRECTION ( 'NONE',  ( -1.000000000000000000, 3.061616997868382648E-16, 0.000000000000000000 ) ) ;
#37244=AXIS2_PLACEMENT_3D ( 'NONE', #63977, #52683, #6818 ) ;
#37246=EDGE_LOOP ( 'NONE', ( #45527, #11393, #33863, #435 ) ) ;
#37349=EDGE_CURVE ( 'NONE', #70803, #43515, #6194, .T. ) ;
#37363=ORIENTED_EDGE ( 'NONE', *, *, #71182, .T. ) ;
#37419=MANIFOLD_SOLID_BREP ( 'Boss-Extrude3', #2035 ) ;
#37500=CARTESIAN_POINT ( 'NONE',  ( 0.000000000000000000, 0.000000000000000000, -175.0000000000000000 ) ) ;
#37541=ORIENTED_EDGE ( 'NONE', *, *, #64442, .F. ) ;
#37559=CARTESIAN_POINT ( 'NONE',  ( 52.50000000000002132, 7.041719095097282063E-15, -175.0000000000000000 ) ) ;
#37604=ADVANCED_FACE ( 'NONE', ( #48619 ), #14402, .F. ) ;
#37636=ORIENTED_EDGE ( 'NONE', *, *, #63123, .T. ) ;
#37750=CARTESIAN_POINT ( 'NONE',  ( -7.500000000000015099, -73.00000000000001421, -204.9999999999999716 ) ) ;
#37805=AXIS2_PLACEMENT_3D ( 'NONE', #39778, #11552, #11195 ) ;
#37827=ORIENTED_EDGE ( 'NONE', *, *, #45504, .T. ) ;
#37842=ORIENTED_EDGE ( 'NONE', *, *, #31568, .T. ) ;
#37883=VECTOR ( 'NONE', #41822, 1000.000000000000000 ) ;
#37913=SURFACE_SIDE_STYLE ('',( #13848 ) ) ;
#38230=CARTESIAN_POINT ( 'NONE',  ( 57.50000000000000000, 7.041719095097280485E-15, -270.0000000000000000 ) ) ;
#38233=DIRECTION ( 'NONE',  ( 1.000000000000000000, 0.000000000000000000, -0.000000000000000000 ) ) ;
#38252=DIRECTION ( 'NONE',  ( -1.000000000000000000, 0.000000000000000000, -0.000000000000000000 ) ) ;
#38410=CARTESIAN_POINT ( 'NONE',  ( 0.000000000000000000, 0.000000000000000000, -175.0000000000000000 ) ) ;
#38426=LINE ( 'NONE', #49684, #34545 ) ;
#38431=AXIS2_PLACEMENT_3D ( 'NONE', #37750, #61424, #49745 ) ;
#38471=CARTESIAN_POINT ( 'NONE',  ( -6.782329983125270800, 10.49999999999999467, -145.0000000000000000 ) ) ;
#38607=VECTOR ( 'NONE', #28516, 1000.000000000000000 ) ;
#38669=CIRCLE ( 'NONE', #39857, 3.299999999999983391 ) ;
#38771=EDGE_LOOP ( 'NONE', ( #14414, #32930, #71803, #72298, #13872, #61340, #36226, #68229 ) ) ;
#38977=FACE_OUTER_BOUND ( 'NONE', #69606, .T. ) ;
#39098=ORIENTED_EDGE ( 'NONE', *, *, #62837, .T. ) ;
#39152=AXIS2_PLACEMENT_3D ( 'NONE', #17760, #64013, #52339 ) ;
#39261=VERTEX_POINT ( 'NONE', #69797 ) ;
#39315=DIRECTION ( 'NONE',  ( -1.000000000000000000, 3.061616997868382648E-16, 0.000000000000000000 ) ) ;
#39359=FACE_OUTER_BOUND ( 'NONE', #31833, .T. ) ;
#39385=AXIS2_PLACEMENT_3D ( 'NONE', #63072, #73946, #45397 ) ;
#39541=VECTOR ( 'NONE', #65089, 1000.000000000000000 ) ;
#39601=DIRECTION ( 'NONE',  ( -2.628368902995175337E-16, -1.000000000000000000, 0.000000000000000000 ) ) ;
#39778=CARTESIAN_POINT ( 'NONE',  ( -7.499999999999969802, 73.00000000000001421, -204.9999999999999716 ) ) ;
#39816=CIRCLE ( 'NONE', #5052, 5.000000000000004441 ) ;
#39857=AXIS2_PLACEMENT_3D ( 'NONE', #50195, #39315, #16373 ) ;
#39904=CARTESIAN_POINT ( 'NONE',  ( 0.000000000000000000, 0.000000000000000000, -145.0000000000000000 ) ) ;
#39917=ORIENTED_EDGE ( 'NONE', *, *, #53796, .T. ) ;
#39974=EDGE_CURVE ( 'NONE', #43515, #40791, #43299, .T. ) ;
#40094=DIRECTION ( 'NONE',  ( -0.000000000000000000, -0.000000000000000000, -1.000000000000000000 ) ) ;
#40140=FACE_OUTER_BOUND ( 'NONE', #66120, .T. ) ;
#40244=VECTOR ( 'NONE', #25752, 1000.000000000000000 ) ;
#40345=DIRECTION ( 'NONE',  ( 1.000000000000000000, -3.061616997868382648E-16, -0.000000000000000000 ) ) ;
#40415=CARTESIAN_POINT ( 'NONE',  ( -7.500000000000016875, -80.00000000000001421, -269.9999999999999432 ) ) ;
#40539=VERTEX_POINT ( 'NONE', #72484 ) ;
#40541=VERTEX_POINT ( 'NONE', #37559 ) ;
#40573=ADVANCED_FACE ( 'NONE', ( #73971 ), #46158, .T. ) ;
#40791=VERTEX_POINT ( 'NONE', #70931 ) ;
#40915=LINE ( 'NONE', #7797, #30520 ) ;
#40932=FACE_OUTER_BOUND ( 'NONE', #47786, .T. ) ;
#41089=VERTEX_POINT ( 'NONE', #22799 ) ;
#41096=LINE ( 'NONE', #17773, #60247 ) ;
#41132=( GEOMETRIC_REPRESENTATION_CONTEXT ( 3 ) GLOBAL_UNCERTAINTY_ASSIGNED_CONTEXT ( ( #10867 ) ) GLOBAL_UNIT_ASSIGNED_CONTEXT ( ( #72476, #60121, #8603 ) ) REPRESENTATION_CONTEXT ( 'NONE', 'WORKASPACE' ) );
#41272=ORIENTED_EDGE ( 'NONE', *, *, #72617, .T. ) ;
#41335=CYLINDRICAL_SURFACE ( 'NONE', #56917, 3.299999999999983391 ) ;
#41357=PLANE ( 'NONE',  #21702 ) ;
#41393=EDGE_LOOP ( 'NONE', ( #4760, #45805, #61030, #36522 ) ) ;
#41518=ORIENTED_EDGE ( 'NONE', *, *, #7454, .F. ) ;
#41588=CARTESIAN_POINT ( 'NONE',  ( -7.500000000000015099, -73.00000000000001421, -204.9999999999999716 ) ) ;
#41791=VERTEX_POINT ( 'NONE', #24537 ) ;
#41822=DIRECTION ( 'NONE',  ( 1.000000000000000000, -3.061616997868382648E-16, -0.000000000000000000 ) ) ;
#41836=DIRECTION ( 'NONE',  ( -1.000000000000000000, 3.061616997868382648E-16, 0.000000000000000000 ) ) ;
#41903=AXIS2_PLACEMENT_3D ( 'NONE', #14969, #49546, #4452 ) ;
#42095=ADVANCED_FACE ( 'NONE', ( #66969 ), #15467, .T. ) ;
#42109=ORIENTED_EDGE ( 'NONE', *, *, #57755, .F. ) ;
#42150=DIRECTION ( 'NONE',  ( 1.000000000000000000, -3.061616997868382648E-16, -0.000000000000000000 ) ) ;
#42422=EDGE_CURVE ( 'NONE', #53797, #70803, #43058, .T. ) ;
#42434=CARTESIAN_POINT ( 'NONE',  ( -57.50000000000000000, 0.000000000000000000, -275.0000000000000000 ) ) ;
#42486=DIRECTION ( 'NONE',  ( -2.628368902995164490E-16, -1.000000000000000000, 0.000000000000000000 ) ) ;
#42668=DIRECTION ( 'NONE',  ( -1.000000000000000000, 0.000000000000000000, 0.000000000000000000 ) ) ;
#42813=PRESENTATION_STYLE_ASSIGNMENT (( #25880 ) ) ;
#43058=LINE ( 'NONE', #65614, #40244 ) ;
#43144=EDGE_CURVE ( 'NONE', #33185, #20050, #38426, .T. ) ;
#43189=CARTESIAN_POINT ( 'NONE',  ( -2.499999999999971578, 69.70000000000001705, -204.9999999999999716 ) ) ;
#43196=ORIENTED_EDGE ( 'NONE', *, *, #50527, .F. ) ;
#43197=ORIENTED_EDGE ( 'NONE', *, *, #19258, .F. ) ;
#43298=ORIENTED_EDGE ( 'NONE', *, *, #67960, .F. ) ;
#43299=LINE ( 'NONE', #55295, #47850 ) ;
#43303=CIRCLE ( 'NONE', #46888, 12.49999999999999645 ) ;
#43315=DIRECTION ( 'NONE',  ( -2.628368902995164490E-16, -1.000000000000000000, 0.000000000000000000 ) ) ;
#43337=FACE_BOUND ( 'NONE', #60193, .T. ) ;
#43395=AXIS2_PLACEMENT_3D ( 'NONE', #48320, #71232, #19735 ) ;
#43405=CIRCLE ( 'NONE', #30329, 3.299999999999983391 ) ;
#43406=PLANE ( 'NONE',  #61763 ) ;
#43420=DIRECTION ( 'NONE',  ( 1.000000000000000000, -3.061616997868382648E-16, -0.000000000000000000 ) ) ;
#43428=ORIENTED_EDGE ( 'NONE', *, *, #54640, .T. ) ;
#43472=VECTOR ( 'NONE', #56190, 1000.000000000000000 ) ;
#43515=VERTEX_POINT ( 'NONE', #71787 ) ;
#43525=PLANE ( 'NONE',  #26089 ) ;
#43547=CARTESIAN_POINT ( 'NONE',  ( 62.50000000000000000, 0.000000000000000000, -275.0000000000000000 ) ) ;
#43554=AXIS2_PLACEMENT_3D ( 'NONE', #68635, #51699, #63009 ) ;
#43696=DIRECTION ( 'NONE',  ( 3.035766082959412415E-16, 1.000000000000000000, 0.000000000000000000 ) ) ;
#44055=EDGE_LOOP ( 'NONE', ( #1101, #37541 ) ) ;
#44087=CARTESIAN_POINT ( 'NONE',  ( 6.782329983125270800, 10.49999999999999467, -125.0000000000000000 ) ) ;
#44228=LINE ( 'NONE', #72767, #9003 ) ;
#44271=VECTOR ( 'NONE', #57316, 1000.000000000000000 ) ;
#44279=CIRCLE ( 'NONE', #38431, 3.299999999999997158 ) ;
#44378=ORIENTED_EDGE ( 'NONE', *, *, #31836, .F. ) ;
#44493=DIRECTION ( 'NONE',  ( 1.000000000000000000, 0.000000000000000000, 0.000000000000000000 ) ) ;
#44539=AXIS2_PLACEMENT_3D ( 'NONE', #56806, #61336, #5681 ) ;
#44718=UNCERTAINTY_MEASURE_WITH_UNIT (LENGTH_MEASURE( 1.000000000000000082E-05 ), #66125, 'distance_accuracy_value', 'NONE');
#44730=( GEOMETRIC_REPRESENTATION_CONTEXT ( 3 ) GLOBAL_UNCERTAINTY_ASSIGNED_CONTEXT ( ( #44718 ) ) GLOBAL_UNIT_ASSIGNED_CONTEXT ( ( #66125, #71729, #8965 ) ) REPRESENTATION_CONTEXT ( 'NONE', 'WORKASPACE' ) );
#44781=VECTOR ( 'NONE', #63339, 1000.000000000000000 ) ;
#44929=ADVANCED_FACE ( 'NONE', ( #5919 ), #17544, .T. ) ;
#45049=DIRECTION ( 'NONE',  ( 1.000000000000000000, 0.000000000000000000, 0.000000000000000000 ) ) ;
#45157=VERTEX_POINT ( 'NONE', #44087 ) ;
#45279=ORIENTED_EDGE ( 'NONE', *, *, #21996, .F. ) ;
#45312=CARTESIAN_POINT ( 'NONE',  ( -2.500000000000014655, -69.70000000000001705, -204.9999999999999716 ) ) ;
#45373=ADVANCED_FACE ( 'NONE', ( #74130 ), #33630, .T. ) ;
#45397=DIRECTION ( 'NONE',  ( -2.628368902995164490E-16, -1.000000000000000000, 0.000000000000000000 ) ) ;
#45421=EDGE_CURVE ( 'NONE', #54824, #56357, #19206, .T. ) ;
#45473=FACE_BOUND ( 'NONE', #6743, .T. ) ;
#45504=EDGE_CURVE ( 'NONE', #62152, #36870, #30478, .T. ) ;
#45527=ORIENTED_EDGE ( 'NONE', *, *, #17612, .F. ) ;
#45541=ORIENTED_EDGE ( 'NONE', *, *, #30194, .T. ) ;
#45676=DIRECTION ( 'NONE',  ( -0.000000000000000000, -0.000000000000000000, -1.000000000000000000 ) ) ;
#45805=ORIENTED_EDGE ( 'NONE', *, *, #59533, .F. ) ;
#45891=ORIENTED_EDGE ( 'NONE', *, *, #16152, .F. ) ;
#45911=VERTEX_POINT ( 'NONE', #25800 ) ;
#45937=CARTESIAN_POINT ( 'NONE',  ( 0.000000000000000000, 0.000000000000000000, -270.0000000000000000 ) ) ;
#45939=CARTESIAN_POINT ( 'NONE',  ( 0.000000000000000000, 0.000000000000000000, -125.0000000000000000 ) ) ;
#45948=DIRECTION ( 'NONE',  ( -1.000000000000000000, 0.000000000000000000, 0.000000000000000000 ) ) ;
#46049=EDGE_LOOP ( 'NONE', ( #4113, #66659, #18420, #72413 ) ) ;
#46092=EDGE_CURVE ( 'NONE', #40791, #15499, #64818, .T. ) ;
#46150=ORIENTED_EDGE ( 'NONE', *, *, #8735, .F. ) ;
#46158=CYLINDRICAL_SURFACE ( 'NONE', #73109, 12.49999999999999645 ) ;
#46177=EDGE_CURVE ( 'NONE', #40541, #48516, #18590, .T. ) ;
#46252=VERTEX_POINT ( 'NONE', #40415 ) ;
#46320=ORIENTED_EDGE ( 'NONE', *, *, #46885, .F. ) ;
#46434=ORIENTED_EDGE ( 'NONE', *, *, #13218, .F. ) ;
#46618=EDGE_CURVE ( 'NONE', #41791, #28195, #26431, .T. ) ;
#46649=LINE ( 'NONE', #68854, #31028 ) ;
#46651=VECTOR ( 'NONE', #48725, 1000.000000000000000 ) ;
#46734=CARTESIAN_POINT ( 'NONE',  ( -7.500000000000016875, -80.00000000000001421, -189.9999999999999147 ) ) ;
#46787=AXIS2_PLACEMENT_3D ( 'NONE', #34034, #56618, #28016 ) ;
#46813=DIRECTION ( 'NONE',  ( 0.7071067811865485719, 8.659560562354946417E-17, -0.7071067811865465735 ) ) ;
#46885=EDGE_CURVE ( 'NONE', #32222, #20050, #34865, .T. ) ;
#46888=AXIS2_PLACEMENT_3D ( 'NONE', #60254, #23523, #24907 ) ;
#47002=FACE_OUTER_BOUND ( 'NONE', #41393, .T. ) ;
#47094=DIRECTION ( 'NONE',  ( -1.000000000000000000, 3.061616997868382648E-16, 0.000000000000000000 ) ) ;
#47263=ADVANCED_FACE ( 'NONE', ( #47002 ), #41357, .F. ) ;
#47724=EDGE_LOOP ( 'NONE', ( #57974, #4846, #43196, #14112 ) ) ;
#47770=CIRCLE ( 'NONE', #56156, 4.999999999999997335 ) ;
#47786=EDGE_LOOP ( 'NONE', ( #10147, #15513, #58052, #15362 ) ) ;
#47843=DIRECTION ( 'NONE',  ( -2.628368902995175337E-16, -1.000000000000000000, 0.000000000000000000 ) ) ;
#47850=VECTOR ( 'NONE', #50006, 1000.000000000000000 ) ;
#47896=AXIS2_PLACEMENT_3D ( 'NONE', #38410, #32749, #50037 ) ;
#48159=ORIENTED_EDGE ( 'NONE', *, *, #28774, .T. ) ;
#48215=AXIS2_PLACEMENT_3D ( 'NONE', #12148, #41836, #35094 ) ;
#48294=LINE ( 'NONE', #30255, #56381 ) ;
#48320=CARTESIAN_POINT ( 'NONE',  ( 0.000000000000000000, 0.000000000000000000, 0.000000000000000000 ) ) ;
#48438=EDGE_CURVE ( 'NONE', #73701, #1246, #15807, .T. ) ;
#48516=VERTEX_POINT ( 'NONE', #5695 ) ;
#48619=FACE_OUTER_BOUND ( 'NONE', #52177, .T. ) ;
#48671=VERTEX_POINT ( 'NONE', #34110 ) ;
#48725=DIRECTION ( 'NONE',  ( -3.035766082959412415E-16, -1.000000000000000000, -0.000000000000000000 ) ) ;
#48736=CARTESIAN_POINT ( 'NONE',  ( -7.500000000000011546, -62.04836822995428491, -189.9999999999999147 ) ) ;
#48895=ORIENTED_EDGE ( 'NONE', *, *, #22866, .F. ) ;
#48946=CYLINDRICAL_SURFACE ( 'NONE', #51253, 3.299999999999997158 ) ;
#49092=ORIENTED_EDGE ( 'NONE', *, *, #54847, .F. ) ;
#49105=CARTESIAN_POINT ( 'NONE',  ( -2.500000000000017319, -80.00000000000001421, -189.9999999999999147 ) ) ;
#49235=CIRCLE ( 'NONE', #3658, 3.299999999999983391 ) ;
#49293=CARTESIAN_POINT ( 'NONE',  ( -2.500000000000015543, -73.00000000000001421, -204.9999999999999716 ) ) ;
#49312=PLANE ( 'NONE',  #7283 ) ;
#49376=AXIS2_PLACEMENT_3D ( 'NONE', #27787, #68764, #5250 ) ;
#49384=CARTESIAN_POINT ( 'NONE',  ( -7.500000000000016875, -80.00000000000001421, -269.9999999999999432 ) ) ;
#49463=EDGE_CURVE ( 'NONE', #28195, #16108, #24821, .T. ) ;
#49492=VECTOR ( 'NONE', #63504, 1000.000000000000000 ) ;
#49546=DIRECTION ( 'NONE',  ( 0.000000000000000000, 0.000000000000000000, -1.000000000000000000 ) ) ;
#49591=DIRECTION ( 'NONE',  ( 1.000000000000000000, -3.061616997868382648E-16, -0.000000000000000000 ) ) ;
#49684=CARTESIAN_POINT ( 'NONE',  ( -7.500000000000015987, -76.30000000000001137, -204.9999999999999716 ) ) ;
#49715=FACE_OUTER_BOUND ( 'NONE', #68991, .T. ) ;
#49745=DIRECTION ( 'NONE',  ( -2.628368902995164490E-16, -1.000000000000000000, 0.000000000000000000 ) ) ;
#49757=LINE ( 'NONE', #55785, #70346 ) ;
#49807=VECTOR ( 'NONE', #50769, 1000.000000000000000 ) ;
#49863=DIRECTION ( 'NONE',  ( -1.000000000000000000, 0.000000000000000000, -0.000000000000000000 ) ) ;
#49875=DIRECTION ( 'NONE',  ( 3.035766082959412415E-16, 1.000000000000000000, 0.000000000000000000 ) ) ;
#49888=ADVANCED_FACE ( 'NONE', ( #1479 ), #64588, .T. ) ;
#49938=CARTESIAN_POINT ( 'NONE',  ( -7.500000000000015987, -76.29999999999999716, -255.0000000000000000 ) ) ;
#49956=CARTESIAN_POINT ( 'NONE',  ( -62.50000000000000000, 0.000000000000000000, -184.9999999999999432 ) ) ;
#49976=PRODUCT ( 'electric motor unit', 'electric motor unit', '', ( #17395 ) ) ;
#50006=DIRECTION ( 'NONE',  ( -3.035766082959412415E-16, -1.000000000000000000, -0.000000000000000000 ) ) ;
#50020=DIRECTION ( 'NONE',  ( -1.000000000000000000, 3.061616997868382648E-16, 0.000000000000000000 ) ) ;
#50025=AXIS2_PLACEMENT_3D ( 'NONE', #57855, #51091, #29618 ) ;
#50037=DIRECTION ( 'NONE',  ( 1.000000000000000000, 0.000000000000000000, 0.000000000000000000 ) ) ;
#50081=EDGE_CURVE ( 'NONE', #48516, #65637, #20847, .T. ) ;
#50195=CARTESIAN_POINT ( 'NONE',  ( -2.499999999999970690, 73.00000000000001421, -255.0000000000000000 ) ) ;
#50303=DIRECTION ( 'NONE',  ( 2.628368902995175337E-16, 1.000000000000000000, 0.000000000000000000 ) ) ;
#50335=LINE ( 'NONE', #49956, #18845 ) ;
#50527=EDGE_CURVE ( 'NONE', #65293, #28744, #61751, .T. ) ;
#50769=DIRECTION ( 'NONE',  ( -0.000000000000000000, -0.000000000000000000, 1.000000000000000000 ) ) ;
#50952=LINE ( 'NONE', #16369, #10575 ) ;
#51091=DIRECTION ( 'NONE',  ( 1.000000000000000000, -3.035766082959412415E-16, 0.000000000000000000 ) ) ;
#51198=ADVANCED_FACE ( 'NONE', ( #68493 ), #35382, .F. ) ;
#51253=AXIS2_PLACEMENT_3D ( 'NONE', #56081, #20393, #54964 ) ;
#51452=CARTESIAN_POINT ( 'NONE',  ( -7.499999999999968914, 79.99999999999998579, -269.9999999999999432 ) ) ;
#51517=CARTESIAN_POINT ( 'NONE',  ( 0.000000000000000000, 0.000000000000000000, -125.0000000000000000 ) ) ;
#51603=AXIS2_PLACEMENT_3D ( 'NONE', #52768, #63695, #55906 ) ;
#51699=DIRECTION ( 'NONE',  ( -1.000000000000000000, 3.061616997868382648E-16, 0.000000000000000000 ) ) ;
#51758=DIRECTION ( 'NONE',  ( -0.000000000000000000, -0.000000000000000000, 1.000000000000000000 ) ) ;
#51765=CARTESIAN_POINT ( 'NONE',  ( -7.500000000000016875, -80.00000000000001421, -269.9999999999999432 ) ) ;
#51977=CARTESIAN_POINT ( 'NONE',  ( -7.499999999999969802, 73.00000000000001421, -255.0000000000000000 ) ) ;
#52177=EDGE_LOOP ( 'NONE', ( #22371, #34774, #37827, #70201 ) ) ;
#52286=CARTESIAN_POINT ( 'NONE',  ( -12.49999999999999645, 1.530808498934191127E-15, -125.0000000000000000 ) ) ;
#52339=DIRECTION ( 'NONE',  ( -1.000000000000000000, 0.000000000000000000, 0.000000000000000000 ) ) ;
#52454=EDGE_CURVE ( 'NONE', #68556, #16557, #850, .T. ) ;
#52529=CARTESIAN_POINT ( 'NONE',  ( -7.500000000000014211, -69.70000000000003126, -255.0000000000000000 ) ) ;
#52574=CIRCLE ( 'NONE', #39385, 3.299999999999997158 ) ;
#52648=EDGE_CURVE ( 'NONE', #48671, #24035, #13556, .T. ) ;
#52655=DIRECTION ( 'NONE',  ( -0.000000000000000000, -0.000000000000000000, -1.000000000000000000 ) ) ;
#52683=DIRECTION ( 'NONE',  ( 0.000000000000000000, 0.000000000000000000, -1.000000000000000000 ) ) ;
#52720=CARTESIAN_POINT ( 'NONE',  ( -2.500000000000016431, -76.30000000000001137, -204.9999999999999716 ) ) ;
#52768=CARTESIAN_POINT ( 'NONE',  ( 0.000000000000000000, 0.000000000000000000, -275.0000000000000000 ) ) ;
#53021=FACE_OUTER_BOUND ( 'NONE', #26652, .T. ) ;
#53057=CIRCLE ( 'NONE', #71015, 62.50000000000000000 ) ;
#53077=LINE ( 'NONE', #65106, #64113 ) ;
#53105=CARTESIAN_POINT ( 'NONE',  ( -2.500000000000011990, -62.44997998398397954, -189.9999999999999147 ) ) ;
#53299=ADVANCED_FACE ( 'NONE', ( #70147 ), #18647, .F. ) ;
#53334=ORIENTED_EDGE ( 'NONE', *, *, #46177, .T. ) ;
#53348=CARTESIAN_POINT ( 'NONE',  ( -2.500000000000017319, -80.00000000000001421, -269.9999999999999432 ) ) ;
#53402=ADVANCED_FACE ( 'NONE', ( #17921 ), #23939, .F. ) ;
#53469=ADVANCED_FACE ( 'NONE', ( #49715 ), #27148, .F. ) ;
#53542=CARTESIAN_POINT ( 'NONE',  ( -2.500000000000017319, -80.00000000000001421, -269.9999999999999432 ) ) ;
#53704=EDGE_LOOP ( 'NONE', ( #59202, #15420, #66240, #31618 ) ) ;
#53711=CARTESIAN_POINT ( 'NONE',  ( -7.499999999999973355, 62.04836822995428491, -275.0000000000000000 ) ) ;
#53758=CARTESIAN_POINT ( 'NONE',  ( -2.499999999999969802, 76.30000000000001137, -204.9999999999999716 ) ) ;
#53796=EDGE_CURVE ( 'NONE', #23489, #40541, #10450, .T. ) ;
#53797=VERTEX_POINT ( 'NONE', #70705 ) ;
#53891=PRESENTATION_STYLE_ASSIGNMENT (( #71160 ) ) ;
#54027=CARTESIAN_POINT ( 'NONE',  ( -7.500000000000016875, -80.00000000000001421, -269.9999999999999432 ) ) ;
#54147=EDGE_CURVE ( 'NONE', #1246, #73701, #27549, .T. ) ;
#54183=DIRECTION ( 'NONE',  ( -0.000000000000000000, -0.000000000000000000, 1.000000000000000000 ) ) ;
#54271=ORIENTED_EDGE ( 'NONE', *, *, #20796, .F. ) ;
#54319=ORIENTED_EDGE ( 'NONE', *, *, #39974, .T. ) ;
#54497=CARTESIAN_POINT ( 'NONE',  ( -2.500000000000015543, -73.00000000000001421, -204.9999999999999716 ) ) ;
#54640=EDGE_CURVE ( 'NONE', #15499, #19508, #39816, .T. ) ;
#54658=DIRECTION ( 'NONE',  ( -0.000000000000000000, -0.000000000000000000, 1.000000000000000000 ) ) ;
#54694=CARTESIAN_POINT ( 'NONE',  ( -6.782329983125270800, 10.49999999999999467, -125.0000000000000000 ) ) ;
#54725=EDGE_CURVE ( 'NONE', #68556, #59175, #53057, .T. ) ;
#54824=VERTEX_POINT ( 'NONE', #48736 ) ;
#54847=EDGE_CURVE ( 'NONE', #70771, #63454, #60408, .T. ) ;
#54930=CARTESIAN_POINT ( 'NONE',  ( -7.500000000000015099, -73.00000000000001421, -255.0000000000000000 ) ) ;
#54964=DIRECTION ( 'NONE',  ( 2.628368902995164490E-16, 1.000000000000000000, 0.000000000000000000 ) ) ;
#55050=DIRECTION ( 'NONE',  ( -1.000000000000000000, 3.061616997868382648E-16, 0.000000000000000000 ) ) ;
#55172=PLANE ( 'NONE',  #13845 ) ;
#55295=CARTESIAN_POINT ( 'NONE',  ( -7.500000000000016875, -80.00000000000001421, -269.9999999999999432 ) ) ;
#55552=CIRCLE ( 'NONE', #43554, 3.299999999999997158 ) ;
#55785=CARTESIAN_POINT ( 'NONE',  ( -7.500000000000014211, -69.70000000000001705, -204.9999999999999716 ) ) ;
#55793=ORIENTED_EDGE ( 'NONE', *, *, #31039, .T. ) ;
#55906=DIRECTION ( 'NONE',  ( -1.000000000000000000, 0.000000000000000000, 0.000000000000000000 ) ) ;
#55982=CARTESIAN_POINT ( 'NONE',  ( -7.499999999999969802, 73.00000000000001421, -255.0000000000000000 ) ) ;
#56081=CARTESIAN_POINT ( 'NONE',  ( -7.499999999999969802, 73.00000000000001421, -204.9999999999999716 ) ) ;
#56156=AXIS2_PLACEMENT_3D ( 'NONE', #38230, #71687, #32582 ) ;
#56190=DIRECTION ( 'NONE',  ( 0.000000000000000000, 0.000000000000000000, -1.000000000000000000 ) ) ;
#56217=EDGE_LOOP ( 'NONE', ( #14164, #36489 ) ) ;
#56357=VERTEX_POINT ( 'NONE', #8926 ) ;
#56381=VECTOR ( 'NONE', #43420, 1000.000000000000000 ) ;
#56539=DIRECTION ( 'NONE',  ( 1.000000000000000000, -3.061616997868382648E-16, -0.000000000000000000 ) ) ;
#56618=DIRECTION ( 'NONE',  ( -0.000000000000000000, -0.000000000000000000, 1.000000000000000000 ) ) ;
#56635=DIRECTION ( 'NONE',  ( -0.000000000000000000, -0.000000000000000000, 1.000000000000000000 ) ) ;
#56806=CARTESIAN_POINT ( 'NONE',  ( -7.500000000000015099, -73.00000000000001421, -255.0000000000000000 ) ) ;
#56843=AXIS2_PLACEMENT_3D ( 'NONE', #22060, #4050, #49875 ) ;
#56917=AXIS2_PLACEMENT_3D ( 'NONE', #6395, #36057, #57898 ) ;
#56965=ORIENTED_EDGE ( 'NONE', *, *, #1428, .F. ) ;
#57316=DIRECTION ( 'NONE',  ( -0.000000000000000000, -0.000000000000000000, -1.000000000000000000 ) ) ;
#57425=ORIENTED_EDGE ( 'NONE', *, *, #21668, .F. ) ;
#57500=AXIS2_PLACEMENT_3D ( 'NONE', #18112, #69965, #34657 ) ;
#57640=ADVANCED_FACE ( 'NONE', ( #62976 ), #70146, .T. ) ;
#57651=CARTESIAN_POINT ( 'NONE',  ( -2.499999999999968914, 79.99999999999998579, -269.9999999999999432 ) ) ;
#57755=EDGE_CURVE ( 'NONE', #28566, #60498, #23380, .T. ) ;
#57810=CARTESIAN_POINT ( 'NONE',  ( 0.000000000000000000, 0.000000000000000000, -175.0000000000000000 ) ) ;
#57855=CARTESIAN_POINT ( 'NONE',  ( -7.499999999999992895, 2.289750019674042456E-15, 0.000000000000000000 ) ) ;
#57898=DIRECTION ( 'NONE',  ( 2.628368902995175337E-16, 1.000000000000000000, 0.000000000000000000 ) ) ;
#57902=ORIENTED_EDGE ( 'NONE', *, *, #13218, .T. ) ;
#57974=ORIENTED_EDGE ( 'NONE', *, *, #67736, .F. ) ;
#58052=ORIENTED_EDGE ( 'NONE', *, *, #60526, .T. ) ;
#58129=ORIENTED_EDGE ( 'NONE', *, *, #48438, .F. ) ;
#58138=ORIENTED_EDGE ( 'NONE', *, *, #3360, .F. ) ;
#58235=EDGE_LOOP ( 'NONE', ( #61573, #62604, #58138, #57425, #43428, #62709 ) ) ;
#58290=ADVANCED_FACE ( 'NONE', ( #27329 ), #55172, .T. ) ;
#58294=DIRECTION ( 'NONE',  ( 0.000000000000000000, 0.000000000000000000, -1.000000000000000000 ) ) ;
#58333=CARTESIAN_POINT ( 'NONE',  ( 0.000000000000000000, 0.000000000000000000, -175.0000000000000000 ) ) ;
#58415=EDGE_CURVE ( 'NONE', #59175, #48516, #20596, .T. ) ;
#58426=ORIENTED_EDGE ( 'NONE', *, *, #73905, .F. ) ;
#58457=CARTESIAN_POINT ( 'NONE',  ( 0.000000000000000000, 0.000000000000000000, -270.0000000000000000 ) ) ;
#58509=DIRECTION ( 'NONE',  ( 0.000000000000000000, -0.000000000000000000, 1.000000000000000000 ) ) ;
#58641=DIRECTION ( 'NONE',  ( 0.000000000000000000, -0.000000000000000000, -1.000000000000000000 ) ) ;
#58897=VERTEX_POINT ( 'NONE', #13320 ) ;
#59046=DIRECTION ( 'NONE',  ( 1.000000000000000000, -3.061616997868382648E-16, -0.000000000000000000 ) ) ;
#59090=DIRECTION ( 'NONE',  ( 1.000000000000000000, -3.061616997868382648E-16, -0.000000000000000000 ) ) ;
#59175=VERTEX_POINT ( 'NONE', #61788 ) ;
#59202=ORIENTED_EDGE ( 'NONE', *, *, #46177, .F. ) ;
#59261=EDGE_CURVE ( 'NONE', #63454, #54824, #71540, .T. ) ;
#59344=LINE ( 'NONE', #9305, #11924 ) ;
#59436=AXIS2_PLACEMENT_3D ( 'NONE', #6550, #24215, #64808 ) ;
#59507=DIRECTION ( 'NONE',  ( -1.000000000000000000, 3.061616997868382648E-16, 0.000000000000000000 ) ) ;
#59517=( GEOMETRIC_REPRESENTATION_CONTEXT ( 3 ) GLOBAL_UNCERTAINTY_ASSIGNED_CONTEXT ( ( #25565 ) ) GLOBAL_UNIT_ASSIGNED_CONTEXT ( ( #13293, #12550, #59539 ) ) REPRESENTATION_CONTEXT ( 'NONE', 'WORKASPACE' ) );
#59533=EDGE_CURVE ( 'NONE', #73701, #45157, #21442, .T. ) ;
#59539=( NAMED_UNIT ( * ) SI_UNIT ( $, .STERADIAN. ) SOLID_ANGLE_UNIT ( ) );
#59567=DIRECTION ( 'NONE',  ( 0.000000000000000000, -0.000000000000000000, 1.000000000000000000 ) ) ;
#59665=DIRECTION ( 'NONE',  ( -0.000000000000000000, -0.000000000000000000, 1.000000000000000000 ) ) ;
#59680=DIRECTION ( 'NONE',  ( 3.035766082959412415E-16, 1.000000000000000000, 0.000000000000000000 ) ) ;
#59697=EDGE_CURVE ( 'NONE', #28744, #39261, #31832, .T. ) ;
#59813=CARTESIAN_POINT ( 'NONE',  ( -7.500000000000011546, -62.04836822995428491, -275.0000000000000000 ) ) ;
#59829=VECTOR ( 'NONE', #71666, 1000.000000000000000 ) ;
#59850=VERTEX_POINT ( 'NONE', #8895 ) ;
#59869=CIRCLE ( 'NONE', #57500, 3.299999999999983391 ) ;
#59915=FILL_AREA_STYLE_COLOUR ( '', #35513 ) ;
#60112=ADVANCED_FACE ( 'NONE', ( #11844 ), #1941, .T. ) ;
#60121=( NAMED_UNIT ( * ) PLANE_ANGLE_UNIT ( ) SI_UNIT ( $, .RADIAN. ) );
#60158=DIRECTION ( 'NONE',  ( 0.000000000000000000, 0.000000000000000000, -1.000000000000000000 ) ) ;
#60193=EDGE_LOOP ( 'NONE', ( #9822, #23728 ) ) ;
#60247=VECTOR ( 'NONE', #40345, 1000.000000000000000 ) ;
#60254=CARTESIAN_POINT ( 'NONE',  ( 0.000000000000000000, 0.000000000000000000, -175.0000000000000000 ) ) ;
#60311=ORIENTED_EDGE ( 'NONE', *, *, #33439, .T. ) ;
#60360=AXIS2_PLACEMENT_3D ( 'NONE', #65605, #55050, #65238 ) ;
#60408=LINE ( 'NONE', #49105, #23017 ) ;
#60498=VERTEX_POINT ( 'NONE', #10656 ) ;
#60526=EDGE_CURVE ( 'NONE', #41089, #32222, #49757, .T. ) ;
#60592=ORIENTED_EDGE ( 'NONE', *, *, #21996, .T. ) ;
#60602=VERTEX_POINT ( 'NONE', #57651 ) ;
#60629=DIRECTION ( 'NONE',  ( 1.000000000000000000, -3.061616997868382648E-16, -0.000000000000000000 ) ) ;
#60891=CYLINDRICAL_SURFACE ( 'NONE', #13374, 3.299999999999983391 ) ;
#60918=EDGE_LOOP ( 'NONE', ( #12094, #16252, #361, #2277 ) ) ;
#60970=CARTESIAN_POINT ( 'NONE',  ( -2.499999999999992895, 7.589415207398510330E-16, 0.000000000000000000 ) ) ;
#61030=ORIENTED_EDGE ( 'NONE', *, *, #54147, .F. ) ;
#61313=EDGE_LOOP ( 'NONE', ( #20172, #61498, #41518, #16494 ) ) ;
#61336=DIRECTION ( 'NONE',  ( -1.000000000000000000, 3.061616997868382648E-16, 0.000000000000000000 ) ) ;
#61340=ORIENTED_EDGE ( 'NONE', *, *, #23372, .T. ) ;
#61424=DIRECTION ( 'NONE',  ( -1.000000000000000000, 3.061616997868382648E-16, 0.000000000000000000 ) ) ;
#61498=ORIENTED_EDGE ( 'NONE', *, *, #59261, .T. ) ;
#61573=ORIENTED_EDGE ( 'NONE', *, *, #12276, .F. ) ;
#61723=CARTESIAN_POINT ( 'NONE',  ( -12.49999999999999645, 1.530808498934191127E-15, -175.0000000000000000 ) ) ;
#61751=CIRCLE ( 'NONE', #17304, 12.49999999999999645 ) ;
#61763=AXIS2_PLACEMENT_3D ( 'NONE', #49384, #59567, #2822 ) ;
#61766=FACE_BOUND ( 'NONE', #6845, .T. ) ;
#61786=AXIS2_PLACEMENT_3D ( 'NONE', #25158, #69175, #63543 ) ;
#61788=CARTESIAN_POINT ( 'NONE',  ( 62.50000000000000000, 0.000000000000000000, -270.0000000000000000 ) ) ;
#61829=ADVANCED_FACE ( 'NONE', ( #38977, #21673 ), #43525, .F. ) ;
#61913=EDGE_LOOP ( 'NONE', ( #42109, #988, #16486, #5826, #58129, #1540, #37842, #48895 ) ) ;
#62032=CARTESIAN_POINT ( 'NONE',  ( -2.499999999999968914, 79.99999999999998579, -189.9999999999999147 ) ) ;
#62152=VERTEX_POINT ( 'NONE', #35322 ) ;
#62164=ORIENTED_EDGE ( 'NONE', *, *, #49463, .T. ) ;
#62231=EDGE_LOOP ( 'NONE', ( #6670, #44378 ) ) ;
#62270=CARTESIAN_POINT ( 'NONE',  ( 0.000000000000000000, 0.000000000000000000, -175.0000000000000000 ) ) ;
#62604=ORIENTED_EDGE ( 'NONE', *, *, #54725, .F. ) ;
#62660=EDGE_LOOP ( 'NONE', ( #19573, #68042, #69523, #67877 ) ) ;
#62709=ORIENTED_EDGE ( 'NONE', *, *, #27823, .F. ) ;
#62718=STYLED_ITEM ( 'NONE', ( #42813 ), #21132 ) ;
#62756=EDGE_CURVE ( 'NONE', #56357, #46252, #3266, .T. ) ;
#62837=EDGE_CURVE ( 'NONE', #60602, #40539, #50952, .T. ) ;
#62976=FACE_OUTER_BOUND ( 'NONE', #37095, .T. ) ;
#63009=DIRECTION ( 'NONE',  ( -2.628368902995164490E-16, -1.000000000000000000, 0.000000000000000000 ) ) ;
#63072=CARTESIAN_POINT ( 'NONE',  ( -7.499999999999969802, 73.00000000000001421, -204.9999999999999716 ) ) ;
#63123=EDGE_CURVE ( 'NONE', #16557, #70771, #7679, .T. ) ;
#63294=LINE ( 'NONE', #46734, #37883 ) ;
#63339=DIRECTION ( 'NONE',  ( -0.000000000000000000, -0.000000000000000000, 1.000000000000000000 ) ) ;
#63386=EDGE_LOOP ( 'NONE', ( #31984, #12671, #45279, #67779 ) ) ;
#63454=VERTEX_POINT ( 'NONE', #53105 ) ;
#63455=DIRECTION ( 'NONE',  ( -0.000000000000000000, -0.000000000000000000, 1.000000000000000000 ) ) ;
#63504=DIRECTION ( 'NONE',  ( -0.000000000000000000, -0.000000000000000000, 1.000000000000000000 ) ) ;
#63543=DIRECTION ( 'NONE',  ( -1.000000000000000000, 0.000000000000000000, 0.000000000000000000 ) ) ;
#63579=DIRECTION ( 'NONE',  ( 1.000000000000000000, 0.000000000000000000, 0.000000000000000000 ) ) ;
#63591=DIRECTION ( 'NONE',  ( -0.000000000000000000, -0.000000000000000000, 1.000000000000000000 ) ) ;
#63646=AXIS2_PLACEMENT_3D ( 'NONE', #51977, #47094, #39601 ) ;
#63695=DIRECTION ( 'NONE',  ( 0.000000000000000000, 0.000000000000000000, -1.000000000000000000 ) ) ;
#63793=CIRCLE ( 'NONE', #49376, 3.299999999999983391 ) ;
#63859=EDGE_LOOP ( 'NONE', ( #8418, #30931, #46320, #5589 ) ) ;
#63872=ADVANCED_FACE ( 'NONE', ( #53021 ), #14261, .F. ) ;
#63945=MECHANICAL_DESIGN_GEOMETRIC_PRESENTATION_REPRESENTATION('',(#62718),#44730);
#63977=CARTESIAN_POINT ( 'NONE',  ( 0.000000000000000000, 0.000000000000000000, -270.0000000000000000 ) ) ;
#64013=DIRECTION ( 'NONE',  ( 0.000000000000000000, 0.000000000000000000, -1.000000000000000000 ) ) ;
#64113=VECTOR ( 'NONE', #59090, 1000.000000000000000 ) ;
#64118=DIRECTION ( 'NONE',  ( 0.000000000000000000, 0.000000000000000000, -1.000000000000000000 ) ) ;
#64239=DIRECTION ( 'NONE',  ( -1.000000000000000000, 3.061616997868382648E-16, 0.000000000000000000 ) ) ;
#64285=ORIENTED_EDGE ( 'NONE', *, *, #31836, .T. ) ;
#64442=EDGE_CURVE ( 'NONE', #33185, #41089, #44279, .T. ) ;
#64588=PLANE ( 'NONE',  #67592 ) ;
#64679=CARTESIAN_POINT ( 'NONE',  ( -7.499999999999969802, 76.29999999999999716, -255.0000000000000000 ) ) ;
#64808=DIRECTION ( 'NONE',  ( -1.000000000000000000, 0.000000000000000000, 0.000000000000000000 ) ) ;
#64809=CIRCLE ( 'NONE', #32365, 62.50000000000000000 ) ;
#64818=CIRCLE ( 'NONE', #46787, 62.50000000000000000 ) ;
#64905=DIRECTION ( 'NONE',  ( 2.628368902995164490E-16, 1.000000000000000000, 0.000000000000000000 ) ) ;
#64960=EDGE_CURVE ( 'NONE', #59850, #71821, #9442, .T. ) ;
#65011=ORIENTED_EDGE ( 'NONE', *, *, #21668, .T. ) ;
#65072=DIRECTION ( 'NONE',  ( -2.628368902995175337E-16, -1.000000000000000000, 0.000000000000000000 ) ) ;
#65089=DIRECTION ( 'NONE',  ( 3.035766082959412415E-16, 1.000000000000000000, 0.000000000000000000 ) ) ;
#65106=CARTESIAN_POINT ( 'NONE',  ( -7.499999999999970690, 69.70000000000003126, -255.0000000000000000 ) ) ;
#65107=ORIENTED_EDGE ( 'NONE', *, *, #54725, .T. ) ;
#65149=EDGE_CURVE ( 'NONE', #14677, #20502, #8518, .T. ) ;
#65238=DIRECTION ( 'NONE',  ( -2.628368902995164490E-16, -1.000000000000000000, 0.000000000000000000 ) ) ;
#65274=ORIENTED_EDGE ( 'NONE', *, *, #52648, .F. ) ;
#65293=VERTEX_POINT ( 'NONE', #29683 ) ;
#65382=CIRCLE ( 'NONE', #61786, 62.50000000000000000 ) ;
#65605=CARTESIAN_POINT ( 'NONE',  ( -7.499999999999969802, 73.00000000000001421, -204.9999999999999716 ) ) ;
#65614=CARTESIAN_POINT ( 'NONE',  ( -7.500000000000016875, -80.00000000000001421, -189.9999999999999147 ) ) ;
#65637=VERTEX_POINT ( 'NONE', #11575 ) ;
#66014=AXIS2_PLACEMENT_3D ( 'NONE', #11528, #51758, #67571 ) ;
#66120=EDGE_LOOP ( 'NONE', ( #65274, #64285, #70003, #58426 ) ) ;
#66125=( LENGTH_UNIT ( ) NAMED_UNIT ( * ) SI_UNIT ( .MILLI., .METRE. ) );
#66217=ORIENTED_EDGE ( 'NONE', *, *, #37349, .T. ) ;
#66240=ORIENTED_EDGE ( 'NONE', *, *, #68842, .T. ) ;
#66465=DIRECTION ( 'NONE',  ( -0.000000000000000000, -0.000000000000000000, 1.000000000000000000 ) ) ;
#66490=FILL_AREA_STYLE_COLOUR ( '', #2728 ) ;
#66658=DIRECTION ( 'NONE',  ( -3.061616997868382648E-16, -1.000000000000000000, 0.000000000000000000 ) ) ;
#66659=ORIENTED_EDGE ( 'NONE', *, *, #65149, .T. ) ;
#66739=CIRCLE ( 'NONE', #27108, 12.49999999999999645 ) ;
#66883=CARTESIAN_POINT ( 'NONE',  ( 0.000000000000000000, 0.000000000000000000, -275.0000000000000000 ) ) ;
#66969=FACE_OUTER_BOUND ( 'NONE', #37246, .T. ) ;
#67192=FACE_OUTER_BOUND ( 'NONE', #18974, .T. ) ;
#67571=DIRECTION ( 'NONE',  ( 1.000000000000000000, 0.000000000000000000, 0.000000000000000000 ) ) ;
#67592=AXIS2_PLACEMENT_3D ( 'NONE', #36749, #32206, #38233 ) ;
#67735=AXIS2_PLACEMENT_3D ( 'NONE', #12691, #8162, #1100 ) ;
#67736=EDGE_CURVE ( 'NONE', #39261, #45157, #36656, .T. ) ;
#67779=ORIENTED_EDGE ( 'NONE', *, *, #49463, .F. ) ;
#67821=DIRECTION ( 'NONE',  ( -1.000000000000000000, 0.000000000000000000, 0.000000000000000000 ) ) ;
#67877=ORIENTED_EDGE ( 'NONE', *, *, #45504, .F. ) ;
#67901=LINE ( 'NONE', #16391, #6210 ) ;
#67960=EDGE_CURVE ( 'NONE', #20502, #58897, #3953, .T. ) ;
#67978=VERTEX_POINT ( 'NONE', #6891 ) ;
#68042=ORIENTED_EDGE ( 'NONE', *, *, #62837, .F. ) ;
#68229=ORIENTED_EDGE ( 'NONE', *, *, #33439, .F. ) ;
#68396=LINE ( 'NONE', #51452, #38607 ) ;
#68493=FACE_OUTER_BOUND ( 'NONE', #47724, .T. ) ;
#68556=VERTEX_POINT ( 'NONE', #20152 ) ;
#68635=CARTESIAN_POINT ( 'NONE',  ( -2.499999999999970690, 73.00000000000001421, -204.9999999999999716 ) ) ;
#68636=CARTESIAN_POINT ( 'NONE',  ( 57.50000000000000000, 7.347880794884118356E-15, -275.0000000000000000 ) ) ;
#68728=CIRCLE ( 'NONE', #18314, 62.50000000000000000 ) ;
#68764=DIRECTION ( 'NONE',  ( -1.000000000000000000, 3.061616997868382648E-16, 0.000000000000000000 ) ) ;
#68842=EDGE_CURVE ( 'NONE', #23489, #65637, #50335, .T. ) ;
#68854=CARTESIAN_POINT ( 'NONE',  ( -2.499999999999968914, 79.99999999999998579, -269.9999999999999432 ) ) ;
#68861=DIRECTION ( 'NONE',  ( -0.000000000000000000, -0.000000000000000000, 1.000000000000000000 ) ) ;
#68873=CARTESIAN_POINT ( 'NONE',  ( -2.500000000000017319, -80.00000000000001421, -269.9999999999999432 ) ) ;
#68991=EDGE_LOOP ( 'NONE', ( #48159, #16239, #22705, #20568 ) ) ;
#69131=AXIS2_PLACEMENT_3D ( 'NONE', #71533, #73755, #28635 ) ;
#69175=DIRECTION ( 'NONE',  ( -0.000000000000000000, -0.000000000000000000, 1.000000000000000000 ) ) ;
#69492=PLANE ( 'NONE',  #50025 ) ;
#69523=ORIENTED_EDGE ( 'NONE', *, *, #28774, .F. ) ;
#69592=DIRECTION ( 'NONE',  ( 0.000000000000000000, 0.000000000000000000, -1.000000000000000000 ) ) ;
#69606=EDGE_LOOP ( 'NONE', ( #39917, #41272 ) ) ;
#69797=CARTESIAN_POINT ( 'NONE',  ( -6.782329983125270800, 10.49999999999999467, -125.0000000000000000 ) ) ;
#69814=CARTESIAN_POINT ( 'NONE',  ( 0.000000000000000000, 0.000000000000000000, -270.0000000000000000 ) ) ;
#69850=CARTESIAN_POINT ( 'NONE',  ( -2.500000000000016431, -76.29999999999999716, -255.0000000000000000 ) ) ;
#69965=DIRECTION ( 'NONE',  ( -1.000000000000000000, 3.061616997868382648E-16, 0.000000000000000000 ) ) ;
#70003=ORIENTED_EDGE ( 'NONE', *, *, #64960, .T. ) ;
#70146=CONICAL_SURFACE ( 'NONE', #5361, 62.50000000000000000, 0.7853981633974497223 ) ;
#70147=FACE_OUTER_BOUND ( 'NONE', #63859, .T. ) ;
#70201=ORIENTED_EDGE ( 'NONE', *, *, #3990, .F. ) ;
#70346=VECTOR ( 'NONE', #56539, 1000.000000000000000 ) ;
#70477=DIRECTION ( 'NONE',  ( 1.000000000000000000, 0.000000000000000000, 0.000000000000000000 ) ) ;
#70548=ORIENTED_EDGE ( 'NONE', *, *, #8755, .T. ) ;
#70649=DIRECTION ( 'NONE',  ( 3.061616997868382648E-16, 1.000000000000000000, -0.000000000000000000 ) ) ;
#70705=CARTESIAN_POINT ( 'NONE',  ( -7.499999999999973355, 62.04836822995428491, -189.9999999999999147 ) ) ;
#70771=VERTEX_POINT ( 'NONE', #31582 ) ;
#70803=VERTEX_POINT ( 'NONE', #27802 ) ;
#70931=CARTESIAN_POINT ( 'NONE',  ( -7.499999999999973355, 62.04836822995428491, -269.9999999999999432 ) ) ;
#71015=AXIS2_PLACEMENT_3D ( 'NONE', #69814, #18316, #1812 ) ;
#71160=SURFACE_STYLE_USAGE ( .BOTH. , #8026 ) ;
#71182=EDGE_CURVE ( 'NONE', #14677, #8861, #59344, .T. ) ;
#71232=DIRECTION ( 'NONE',  ( 0.000000000000000000, 0.000000000000000000, 1.000000000000000000 ) ) ;
#71272=CARTESIAN_POINT ( 'NONE',  ( -7.500000000000016875, -80.00000000000001421, -269.9999999999999432 ) ) ;
#71334=DIRECTION ( 'NONE',  ( 1.000000000000000000, -3.061616997868382648E-16, -0.000000000000000000 ) ) ;
#71533=CARTESIAN_POINT ( 'NONE',  ( -7.500000000000016875, -80.00000000000001421, -189.9999999999999147 ) ) ;
#71540=CIRCLE ( 'NONE', #39152, 62.50000000000000000 ) ;
#71626=EDGE_CURVE ( 'NONE', #53797, #62152, #64809, .T. ) ;
#71666=DIRECTION ( 'NONE',  ( 0.000000000000000000, 0.000000000000000000, 1.000000000000000000 ) ) ;
#71687=DIRECTION ( 'NONE',  ( -1.224646799147353207E-16, 1.000000000000000000, 0.000000000000000000 ) ) ;
#71692=DIRECTION ( 'NONE',  ( -1.000000000000000000, 3.061616997868382648E-16, 0.000000000000000000 ) ) ;
#71729=( NAMED_UNIT ( * ) PLANE_ANGLE_UNIT ( ) SI_UNIT ( $, .RADIAN. ) );
#71787=CARTESIAN_POINT ( 'NONE',  ( -7.499999999999968914, 79.99999999999998579, -269.9999999999999432 ) ) ;
#71803=ORIENTED_EDGE ( 'NONE', *, *, #11806, .T. ) ;
#71821=VERTEX_POINT ( 'NONE', #53758 ) ;
#72072=FACE_BOUND ( 'NONE', #56217, .T. ) ;
#72082=DIRECTION ( 'NONE',  ( 2.628368902995175337E-16, 1.000000000000000000, 0.000000000000000000 ) ) ;
#72104=FACE_OUTER_BOUND ( 'NONE', #61313, .T. ) ;
#72108=FILL_AREA_STYLE ('',( #66490 ) ) ;
#72298=ORIENTED_EDGE ( 'NONE', *, *, #58415, .F. ) ;
#72353=DIRECTION ( 'NONE',  ( 0.000000000000000000, 0.000000000000000000, -1.000000000000000000 ) ) ;
#72413=ORIENTED_EDGE ( 'NONE', *, *, #30270, .F. ) ;
#72476=( LENGTH_UNIT ( ) NAMED_UNIT ( * ) SI_UNIT ( .MILLI., .METRE. ) );
#72484=CARTESIAN_POINT ( 'NONE',  ( -2.499999999999974243, 62.44997998398397954, -270.0000000000000000 ) ) ;
#72617=EDGE_CURVE ( 'NONE', #40541, #23489, #28783, .T. ) ;
#72767=CARTESIAN_POINT ( 'NONE',  ( -6.782329983125270800, 10.49999999999999467, -145.0000000000000000 ) ) ;
#72820=SHAPE_REPRESENTATION ( 'electric motor unit', ( #43395 ), #41132 ) ;
#73011=DIRECTION ( 'NONE',  ( 1.000000000000000000, -3.061616997868382648E-16, 0.000000000000000000 ) ) ;
#73109=AXIS2_PLACEMENT_3D ( 'NONE', #57810, #63455, #45049 ) ;
#73193=CARTESIAN_POINT ( 'NONE',  ( -7.500000000000015099, -73.00000000000001421, -255.0000000000000000 ) ) ;
#73322=CARTESIAN_POINT ( 'NONE',  ( 6.782329983125270800, 10.49999999999999467, -145.0000000000000000 ) ) ;
#73390=CARTESIAN_POINT ( 'NONE',  ( -7.499999999999968914, 79.99999999999998579, -269.9999999999999432 ) ) ;
#73395=ORIENTED_EDGE ( 'NONE', *, *, #68842, .F. ) ;
#73542=VECTOR ( 'NONE', #59046, 1000.000000000000000 ) ;
#73629=PRODUCT_DEFINITION_FORMATION_WITH_SPECIFIED_SOURCE ( 'ANY', '', #49976, .NOT_KNOWN. ) ;
#73659=ADVANCED_FACE ( 'NONE', ( #40932 ), #36751, .F. ) ;
#73701=VERTEX_POINT ( 'NONE', #7814 ) ;
#73755=DIRECTION ( 'NONE',  ( 0.000000000000000000, 0.000000000000000000, -1.000000000000000000 ) ) ;
#73905=EDGE_CURVE ( 'NONE', #24035, #71821, #1350, .T. ) ;
#73946=DIRECTION ( 'NONE',  ( -1.000000000000000000, 3.061616997868382648E-16, 0.000000000000000000 ) ) ;
#73971=FACE_OUTER_BOUND ( 'NONE', #61913, .T. ) ;
#74072=ORIENTED_EDGE ( 'NONE', *, *, #30194, .F. ) ;
#74130=FACE_OUTER_BOUND ( 'NONE', #58235, .T. ) ;
#74262=ORIENTED_EDGE ( 'NONE', *, *, #23184, .F. ) ;
#74281=ORIENTED_EDGE ( 'NONE', *, *, #3360, .T. ) ;
#74290=VECTOR ( 'NONE', #25708, 1000.000000000000000 ) ;
ENDSEC;
END-ISO-10303-21;
